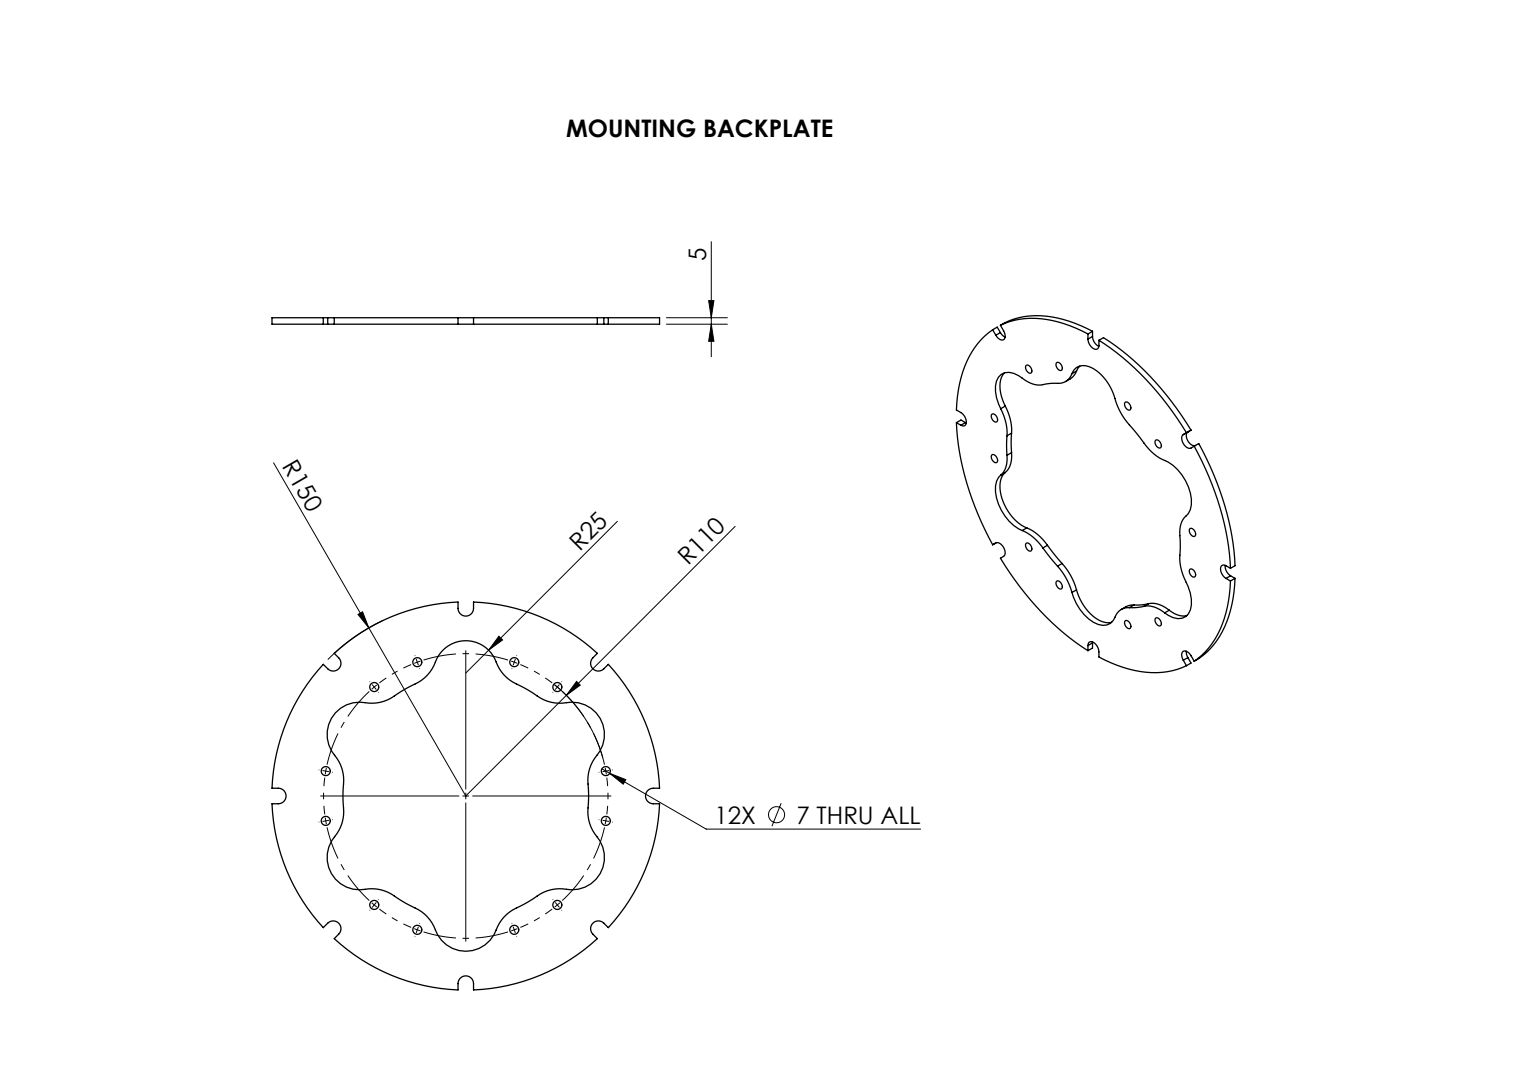
ISO-10303-21;
HEADER;
FILE_DESCRIPTION (('STEP AP214'),
    '1' );
FILE_NAME ('mounting backplate.step',
    '2026-09-21T15:58:29',
    ( '' ),
    ( '' ),
    'SwSTEP 2.0',
    'SolidWorks 2026',
    '' );
FILE_SCHEMA (( 'AUTOMOTIVE_DESIGN' ));
ENDSEC;

DATA;
#3=ORIENTED_EDGE ( 'NONE', *, *, #6672, .T. ) ;
#13=EDGE_CURVE ( 'NONE', #31164, #27343, #2215, .T. ) ;
#22=EDGE_CURVE ( 'NONE', #8678, #8115, #12991, .T. ) ;
#37=CARTESIAN_POINT ( 'NONE',  ( -5.999999999999998224, -145.0000000000000568, 27.50000000000000000 ) ) ;
#40=VERTEX_POINT ( 'NONE', #29073 ) ;
#41=B_SPLINE_CURVE_WITH_KNOTS ( 'NONE', 3,
 ( #1307, #24180, #18746, #30167, #7133, #7874, #14025, #11030, #2597, #10859, #22124, #25848, #25677, #17230, #22672, #5430, #8588, #5792, #22296, #5042, #34557, #25296, #13675, #2430, #10681, #28652, #33922, #25131, #25473, #19674, #2985, #16478, #17025, #14220, #34121 ),
 .UNSPECIFIED., .F., .F.,
 ( 4, 2, 1, 1, 2, 2, 1, 2, 2, 2, 2, 1, 2, 2, 1, 2, 2, 1, 1, 2, 4 ),
 ( 0.05563282717606015532, 0.06778080578355423491, 0.07992878439104830757, 0.1042247416060363280, 0.1163727202135303451, 0.1285206988210243761, 0.1528166560360122717, 0.1771126132510001672, 0.1892605918584941982, 0.2014085704659882570, 0.2500004848959641035, 0.2985923993259401166, 0.3107403779334341754, 0.3228883565409281786, 0.3471843137559161296, 0.3714802709709040252, 0.3836282495783980284, 0.3957762281858920317, 0.4200721854008799272, 0.4322201640083740415, 0.4443681426158681003 ),
 .UNSPECIFIED. ) ;
#42=CARTESIAN_POINT ( 'NONE',  ( -51.68138994340220904, 113.8157894736842053, 27.50000000000000000 ) ) ;
#46=ORIENTED_EDGE ( 'NONE', *, *, #8957, .F. ) ;
#56=DIRECTION ( 'NONE',  ( 1.000000000000000000, 0.000000000000000000, 0.000000000000000000 ) ) ;
#61=FACE_OUTER_BOUND ( 'NONE', #20749, .T. ) ;
#79=DIRECTION ( 'NONE',  ( -0.000000000000000000, -0.000000000000000000, -1.000000000000000000 ) ) ;
#84=FACE_OUTER_BOUND ( 'NONE', #29361, .T. ) ;
#90=DIRECTION ( 'NONE',  ( 0.000000000000000000, 0.000000000000000000, 1.000000000000000000 ) ) ;
#114=VERTEX_POINT ( 'NONE', #394 ) ;
#118=DIRECTION ( 'NONE',  ( -0.7071067811865463515, 0.7071067811865487940, 0.000000000000000000 ) ) ;
#130=ORIENTED_EDGE ( 'NONE', *, *, #1368, .T. ) ;
#139=CARTESIAN_POINT ( 'NONE',  ( 98.28784258492957804, -106.7731239591692116, 32.50000000000000000 ) ) ;
#144=CIRCLE ( 'NONE', #10915, 3.499999999999996003 ) ;
#156=AXIS2_PLACEMENT_3D ( 'NONE', #424, #5891, #17129 ) ;
#188=DIRECTION ( 'NONE',  ( 0.7071067811865512365, 0.7071067811865439090, -0.000000000000000000 ) ) ;
#194=CIRCLE ( 'NONE', #12140, 30.00000000000000000 ) ;
#212=CIRCLE ( 'NONE', #9335, 3.500000000000003109 ) ;
#219=LINE ( 'NONE', #29087, #28624 ) ;
#231=ORIENTED_EDGE ( 'NONE', *, *, #33765, .T. ) ;
#248=ORIENTED_EDGE ( 'NONE', *, *, #1490, .F. ) ;
#250=ORIENTED_EDGE ( 'NONE', *, *, #33993, .T. ) ;
#252=FACE_OUTER_BOUND ( 'NONE', #33217, .T. ) ;
#261=EDGE_CURVE ( 'NONE', #2865, #30153, #36198, .T. ) ;
#273=DIRECTION ( 'NONE',  ( 1.000000000000000000, 0.000000000000000000, 0.000000000000000000 ) ) ;
#277=AXIS2_PLACEMENT_3D ( 'NONE', #26246, #15000, #11980 ) ;
#284=ORIENTED_EDGE ( 'NONE', *, *, #26597, .T. ) ;
#303=DIRECTION ( 'NONE',  ( 0.000000000000000000, 0.000000000000000000, 1.000000000000000000 ) ) ;
#315=ORIENTED_EDGE ( 'NONE', *, *, #9812, .T. ) ;
#343=FILL_AREA_STYLE_COLOUR ( '', #32786 ) ;
#361=CARTESIAN_POINT ( 'NONE',  ( 67.30619744049005249, 84.18124734178236679, 32.50000000000000000 ) ) ;
#375=CARTESIAN_POINT ( 'NONE',  ( -145.0000000000000000, 6.000000000001517009, 32.50000000000000000 ) ) ;
#385=AXIS2_PLACEMENT_3D ( 'NONE', #13978, #33868, #34423 ) ;
#394=CARTESIAN_POINT ( 'NONE',  ( 96.53048327204960799, 102.5304832720492527, 32.50000000000000000 ) ) ;
#412=CARTESIAN_POINT ( 'NONE',  ( -55.27226924886181791, -77.26562141134519379, 27.50000000000000000 ) ) ;
#424=CARTESIAN_POINT ( 'NONE',  ( 0.000000000000000000, 0.000000000000000000, 32.50000000000000000 ) ) ;
#434=CIRCLE ( 'NONE', #22609, 3.500000000000003109 ) ;
#436=CARTESIAN_POINT ( 'NONE',  ( 51.68138994340220904, -113.8157894736842053, 32.50002500000000083 ) ) ;
#440=CARTESIAN_POINT ( 'NONE',  ( -18.19096825468298206, -112.1612438786420256, 32.50000000000000000 ) ) ;
#460=VERTEX_POINT ( 'NONE', #14249 ) ;
#491=CARTESIAN_POINT ( 'NONE',  ( 95.00000000000001421, 0.000000000000000000, 27.50000000000000000 ) ) ;
#492=ORIENTED_EDGE ( 'NONE', *, *, #13456, .T. ) ;
#511=CARTESIAN_POINT ( 'NONE',  ( -6.284666409917640040E-14, -6.000000000000000000, 27.50000000000000000 ) ) ;
#521=AXIS2_PLACEMENT_3D ( 'NONE', #20689, #29495, #32120 ) ;
#525=CARTESIAN_POINT ( 'NONE',  ( 96.53048327204888324, -102.5304832720499633, 27.50000000000000000 ) ) ;
#526=PLANE ( 'NONE',  #25503 ) ;
#527=CARTESIAN_POINT ( 'NONE',  ( 149.8799519615616589, 5.999999999999476863, 32.55002500000000509 ) ) ;
#535=DIRECTION ( 'NONE',  ( 1.000000000000000000, 0.000000000000000000, 0.000000000000000000 ) ) ;
#540=CIRCLE ( 'NONE', #34686, 5.999999999999999112 ) ;
#562=CARTESIAN_POINT ( 'NONE',  ( 82.38629821025696742, 72.56049487126330177, 32.49999999999998579 ) ) ;
#563=DIRECTION ( 'NONE',  ( 0.000000000000000000, 0.000000000000000000, 1.000000000000000000 ) ) ;
#589=FACE_OUTER_BOUND ( 'NONE', #27728, .T. ) ;
#591=ORIENTED_EDGE ( 'NONE', *, *, #22851, .F. ) ;
#613=FACE_OUTER_BOUND ( 'NONE', #23040, .T. ) ;
#615=EDGE_CURVE ( 'NONE', #4570, #3560, #17776, .T. ) ;
#641=CARTESIAN_POINT ( 'NONE',  ( -98.28784258492883907, 106.7731239591698937, 32.50000000000000000 ) ) ;
#643=CYLINDRICAL_SURFACE ( 'NONE', #1498, 30.00000000000000000 ) ;
#646=DIRECTION ( 'NONE',  ( -0.000000000000000000, -0.000000000000000000, 1.000000000000000000 ) ) ;
#653=DIRECTION ( 'NONE',  ( 0.000000000000000000, 0.000000000000000000, 1.000000000000000000 ) ) ;
#654=ADVANCED_FACE ( 'NONE', ( #5002 ), #21520, .F. ) ;
#677=ORIENTED_EDGE ( 'NONE', *, *, #11143, .T. ) ;
#684=EDGE_LOOP ( 'NONE', ( #31991, #3562, #3930, #7996 ) ) ;
#694=CARTESIAN_POINT ( 'NONE',  ( 149.8799519615616589, 5.999999999999476863, 27.50000000000000000 ) ) ;
#711=EDGE_CURVE ( 'NONE', #22882, #22692, #14376, .T. ) ;
#735=CARTESIAN_POINT ( 'NONE',  ( -37.50000000000000000, -103.4105893997321743, 32.50000000000000000 ) ) ;
#738=CARTESIAN_POINT ( 'NONE',  ( 105.8342059669409281, 39.11274920687675660, 32.50000000000000000 ) ) ;
#739=DIRECTION ( 'NONE',  ( 1.000000000000000000, 0.000000000000000000, 0.000000000000000000 ) ) ;
#785=DIRECTION ( 'NONE',  ( -0.000000000000000000, -0.000000000000000000, -1.000000000000000000 ) ) ;
#805=CARTESIAN_POINT ( 'NONE',  ( 2.577124608817066953, -119.9999535335656162, 32.50000000000000000 ) ) ;
#806=EDGE_CURVE ( 'NONE', #8770, #16892, #29355, .T. ) ;
#812=EDGE_CURVE ( 'NONE', #10608, #13259, #17726, .T. ) ;
#813=CYLINDRICAL_SURFACE ( 'NONE', #32755, 30.00000000000000000 ) ;
#815=CARTESIAN_POINT ( 'NONE',  ( -23.49188638668713480, -103.5527587461262442, 32.50001250000000397 ) ) ;
#839=ORIENTED_EDGE ( 'NONE', *, *, #21442, .F. ) ;
#843=PLANE ( 'NONE',  #24821 ) ;
#844=FACE_OUTER_BOUND ( 'NONE', #14924, .T. ) ;
#868=VECTOR ( 'NONE', #29592, 1000.000000000000000 ) ;
#877=CARTESIAN_POINT ( 'NONE',  ( -72.72667006429185221, -101.6652913307173662, 27.50000000000000000 ) ) ;
#891=CARTESIAN_POINT ( 'NONE',  ( -51.68138994340220904, -113.8157894736842053, 32.50002500000000083 ) ) ;
#901=CARTESIAN_POINT ( 'NONE',  ( -94.55012560584668790, 9.234378588655390629, 27.50000000000000000 ) ) ;
#935=ORIENTED_EDGE ( 'NONE', *, *, #19624, .F. ) ;
#938=LINE ( 'NONE', #12358, #6254 ) ;
#941=DIRECTION ( 'NONE',  ( 0.000000000000000000, 0.000000000000000000, 1.000000000000000000 ) ) ;
#963=EDGE_LOOP ( 'NONE', ( #4579, #25349, #35849, #2137 ) ) ;
#976=CYLINDRICAL_SURFACE ( 'NONE', #1827, 3.500000000000003109 ) ;
#986=AXIS2_PLACEMENT_3D ( 'NONE', #19892, #19180, #30599 ) ;
#991=DIRECTION ( 'NONE',  ( 0.000000000000000000, 0.000000000000000000, 1.000000000000000000 ) ) ;
#1012=DIRECTION ( 'NONE',  ( -1.000000000000000000, 0.000000000000000000, 0.000000000000000000 ) ) ;
#1026=VECTOR ( 'NONE', #13351, 1000.000000000000000 ) ;
#1033=LINE ( 'NONE', #12458, #22337 ) ;
#1070=ORIENTED_EDGE ( 'NONE', *, *, #28796, .T. ) ;
#1078=DIRECTION ( 'NONE',  ( 1.000000000000000000, 0.000000000000000000, 0.000000000000000000 ) ) ;
#1080=AXIS2_PLACEMENT_3D ( 'NONE', #23094, #15030, #8849 ) ;
#1098=ORIENTED_EDGE ( 'NONE', *, *, #4957, .T. ) ;
#1100=DIRECTION ( 'NONE',  ( 0.000000000000000000, 0.000000000000000000, 1.000000000000000000 ) ) ;
#1122=CARTESIAN_POINT ( 'NONE',  ( 97.20669606277387231, 67.55917549538906997, 32.49999999999999289 ) ) ;
#1124=CIRCLE ( 'NONE', #13086, 95.00000000000001421 ) ;
#1164=CARTESIAN_POINT ( 'NONE',  ( 4.242640687119292764, 4.242640687119187071, 27.50000000000000000 ) ) ;
#1188=EDGE_LOOP ( 'NONE', ( #33444, #30548, #5664, #10870 ) ) ;
#1196=CYLINDRICAL_SURFACE ( 'NONE', #14748, 3.500000000000003109 ) ;
#1209=ORIENTED_EDGE ( 'NONE', *, *, #23387, .T. ) ;
#1214=CARTESIAN_POINT ( 'NONE',  ( -4.242640687119273224, -4.242640687119226151, 32.50000000000000000 ) ) ;
#1215=VECTOR ( 'NONE', #21555, 1000.000000000000000 ) ;
#1224=VERTEX_POINT ( 'NONE', #20518 ) ;
#1233=DIRECTION ( 'NONE',  ( 1.000000000000000000, 0.000000000000000000, 0.000000000000000000 ) ) ;
#1238=ORIENTED_EDGE ( 'NONE', *, *, #28621, .T. ) ;
#1262=CARTESIAN_POINT ( 'NONE',  ( 0.000000000000000000, 95.00000000000001421, 32.50000000000000000 ) ) ;
#1293=CARTESIAN_POINT ( 'NONE',  ( 51.68138994340220904, 113.8157894736842053, 27.50000000000000000 ) ) ;
#1294=AXIS2_PLACEMENT_3D ( 'NONE', #11887, #20153, #8708 ) ;
#1297=EDGE_LOOP ( 'NONE', ( #315, #8437, #30494, #23979 ) ) ;
#1305=DIRECTION ( 'NONE',  ( 0.000000000000000000, 0.000000000000000000, 1.000000000000000000 ) ) ;
#1307=CARTESIAN_POINT ( 'NONE',  ( 101.4252494179806661, -31.43181965332042438, 32.50001250000000397 ) ) ;
#1308=CARTESIAN_POINT ( 'NONE',  ( -37.50000000000000000, 103.4105893997321743, 32.50000000000000000 ) ) ;
#1355=DIRECTION ( 'NONE',  ( -0.000000000000000000, -0.000000000000000000, -1.000000000000000000 ) ) ;
#1358=VERTEX_POINT ( 'NONE', #15276 ) ;
#1368=EDGE_CURVE ( 'NONE', #28369, #25631, #212, .T. ) ;
#1381=CARTESIAN_POINT ( 'NONE',  ( 124.4080600076931375, 12.15049814296589226, 32.50000000000000000 ) ) ;
#1388=DIRECTION ( 'NONE',  ( -1.000000000000000000, 0.000000000000000000, 0.000000000000000000 ) ) ;
#1391=EDGE_CURVE ( 'NONE', #4682, #26755, #18090, .T. ) ;
#1398=ORIENTED_EDGE ( 'NONE', *, *, #1368, .F. ) ;
#1400=DIRECTION ( 'NONE',  ( -0.000000000000000000, -0.000000000000000000, 1.000000000000000000 ) ) ;
#1403=EDGE_CURVE ( 'NONE', #8057, #11432, #1033, .T. ) ;
#1422=PRODUCT_CONTEXT ( 'NONE', #17085, 'mechanical' ) ;
#1429=DIRECTION ( 'NONE',  ( 0.000000000000000000, 0.000000000000000000, 1.000000000000000000 ) ) ;
#1442=VERTEX_POINT ( 'NONE', #16390 ) ;
#1456=CIRCLE ( 'NONE', #277, 3.499999999999996003 ) ;
#1458=EDGE_LOOP ( 'NONE', ( #32965, #6091, #32772, #35012 ) ) ;
#1490=EDGE_CURVE ( 'NONE', #35726, #27793, #15131, .T. ) ;
#1498=AXIS2_PLACEMENT_3D ( 'NONE', #17511, #11883, #32492 ) ;
#1567=EDGE_CURVE ( 'NONE', #4390, #26755, #33266, .T. ) ;
#1589=CYLINDRICAL_SURFACE ( 'NONE', #32182, 3.500000000000003109 ) ;
#1598=VERTEX_POINT ( 'NONE', #5514 ) ;
#1604=CARTESIAN_POINT ( 'NONE',  ( -108.3061974404900241, -19.22934205794863516, 27.50000000000000000 ) ) ;
#1605=CARTESIAN_POINT ( 'NONE',  ( 4.242640687119310527, 4.242640687119267007, 32.50000000000000000 ) ) ;
#1607=EDGE_CURVE ( 'NONE', #14541, #13732, #10344, .T. ) ;
#1609=FACE_OUTER_BOUND ( 'NONE', #3806, .T. ) ;
#1613=DIRECTION ( 'NONE',  ( 1.000000000000000000, 0.000000000000000000, 0.000000000000000000 ) ) ;
#1617=CARTESIAN_POINT ( 'NONE',  ( 101.7384897088151234, 110.2237710830533217, 32.50000000000000000 ) ) ;
#1624=ORIENTED_EDGE ( 'NONE', *, *, #19700, .T. ) ;
#1636=ADVANCED_FACE ( 'NONE', ( #19937 ), #2690, .F. ) ;
#1641=AXIS2_PLACEMENT_3D ( 'NONE', #16254, #4438, #15690 ) ;
#1643=ORIENTED_EDGE ( 'NONE', *, *, #12876, .F. ) ;
#1657=ORIENTED_EDGE ( 'NONE', *, *, #3901, .F. ) ;
#1660=AXIS2_PLACEMENT_3D ( 'NONE', #17232, #31452, #28655 ) ;
#1661=LINE ( 'NONE', #35609, #19441 ) ;
#1667=CARTESIAN_POINT ( 'NONE',  ( -107.0891125874437506, 43.89216747908891136, 32.49999999999999289 ) ) ;
#1673=LINE ( 'NONE', #26984, #868 ) ;
#1677=AXIS2_PLACEMENT_3D ( 'NONE', #27123, #4086, #26955 ) ;
#1692=ORIENTED_EDGE ( 'NONE', *, *, #6728, .T. ) ;
#1706=AXIS2_PLACEMENT_3D ( 'NONE', #9005, #11439, #32023 ) ;
#1712=CARTESIAN_POINT ( 'NONE',  ( -67.30619744049063513, -84.18124734178186941, 27.50000000000000000 ) ) ;
#1739=CARTESIAN_POINT ( 'NONE',  ( -103.1837590831665210, -33.77668192579397299, 32.49999999999999289 ) ) ;
#1760=DIRECTION ( 'NONE',  ( -0.000000000000000000, -0.000000000000000000, -1.000000000000000000 ) ) ;
#1767=ORIENTED_EDGE ( 'NONE', *, *, #6528, .F. ) ;
#1768=CYLINDRICAL_SURFACE ( 'NONE', #23835, 95.00000000000001421 ) ;
#1784=ORIENTED_EDGE ( 'NONE', *, *, #22476, .T. ) ;
#1786=CARTESIAN_POINT ( 'NONE',  ( -145.0000000000000568, 1.518182058997189877E-12, 32.55002500000000509 ) ) ;
#1787=CARTESIAN_POINT ( 'NONE',  ( 145.0000000000000568, -5.056524707326808249E-13, 32.55002500000000509 ) ) ;
#1809=FACE_OUTER_BOUND ( 'NONE', #29343, .T. ) ;
#1827=AXIS2_PLACEMENT_3D ( 'NONE', #29849, #8087, #1908 ) ;
#1830=CARTESIAN_POINT ( 'NONE',  ( 0.000000000000000000, -95.00000000000001421, 32.50002500000000083 ) ) ;
#1831=CARTESIAN_POINT ( 'NONE',  ( -103.1654841881149025, 61.26096253783315859, 32.50000000000000711 ) ) ;
#1880=ORIENTED_EDGE ( 'NONE', *, *, #6661, .F. ) ;
#1908=DIRECTION ( 'NONE',  ( 1.000000000000000000, 0.000000000000000000, 0.000000000000000000 ) ) ;
#1918=CARTESIAN_POINT ( 'NONE',  ( -107.2777853369584591, -46.05195005975305378, 32.50000000000000000 ) ) ;
#1920=EDGE_LOOP ( 'NONE', ( #8732, #36744, #26794, #12307, #11729, #24164, #19809, #10074, #25151, #33826, #24025, #21911, #12744, #33055, #6237, #10358, #21105, #28122, #28960, #16884, #3124, #8179, #36525, #19792, #28859, #18087, #7295, #250, #22492, #26605, #15987, #18220, #231, #15241, #9497 ) ) ;
#1924=FACE_OUTER_BOUND ( 'NONE', #9242, .T. ) ;
#1932=DIRECTION ( 'NONE',  ( -0.000000000000000000, -0.000000000000000000, -1.000000000000000000 ) ) ;
#1946=VERTEX_POINT ( 'NONE', #36374 ) ;
#1950=EDGE_CURVE ( 'NONE', #13345, #8665, #9606, .T. ) ;
#1952=VERTEX_POINT ( 'NONE', #25297 ) ;
#1961=EDGE_CURVE ( 'NONE', #22389, #3923, #34473, .T. ) ;
#1962=AXIS2_PLACEMENT_3D ( 'NONE', #32236, #34705, #9006 ) ;
#1963=DIRECTION ( 'NONE',  ( 0.000000000000000000, 0.000000000000000000, 1.000000000000000000 ) ) ;
#1972=ADVANCED_FACE ( 'NONE', ( #8779 ), #526, .F. ) ;
#1973=ORIENTED_EDGE ( 'NONE', *, *, #6672, .F. ) ;
#1992=CARTESIAN_POINT ( 'NONE',  ( -111.8061974404900241, -19.22934205794863516, 27.50000000000000000 ) ) ;
#1998=EDGE_CURVE ( 'NONE', #114, #35512, #32055, .T. ) ;
#2006=EDGE_CURVE ( 'NONE', #23321, #6715, #20562, .T. ) ;
#2025=CARTESIAN_POINT ( 'NONE',  ( 72.72667006429044534, -101.6652913307183610, 32.50000000000000000 ) ) ;
#2031=ADVANCED_FACE ( 'NONE', ( #34470 ), #14967, .F. ) ;
#2033=EDGE_LOOP ( 'NONE', ( #19508, #14993, #29571, #36394 ) ) ;
#2049=VERTEX_POINT ( 'NONE', #139 ) ;
#2070=CARTESIAN_POINT ( 'NONE',  ( 23.49154088336464952, -103.5526315789473699, 32.50002500000000083 ) ) ;
#2085=EDGE_CURVE ( 'NONE', #19856, #15010, #11705, .T. ) ;
#2093=CARTESIAN_POINT ( 'NONE',  ( -82.27241335952211898, -47.49999999999924682, 27.50000000000000000 ) ) ;
#2113=LINE ( 'NONE', #10758, #18957 ) ;
#2118=EDGE_LOOP ( 'NONE', ( #28713, #23285, #17247, #29365 ) ) ;
#2119=CARTESIAN_POINT ( 'NONE',  ( 0.000000000000000000, 0.000000000000000000, 27.50000000000000000 ) ) ;
#2126=CIRCLE ( 'NONE', #33260, 30.00000000000001421 ) ;
#2133=CARTESIAN_POINT ( 'NONE',  ( 0.000000000000000000, 0.000000000000000000, 27.50000000000000000 ) ) ;
#2137=ORIENTED_EDGE ( 'NONE', *, *, #34736, .T. ) ;
#2155=DIRECTION ( 'NONE',  ( 0.000000000000000000, 0.000000000000000000, 1.000000000000000000 ) ) ;
#2160=FACE_OUTER_BOUND ( 'NONE', #24834, .T. ) ;
#2184=ORIENTED_EDGE ( 'NONE', *, *, #13444, .F. ) ;
#2203=ORIENTED_EDGE ( 'NONE', *, *, #22583, .F. ) ;
#2212=VECTOR ( 'NONE', #29599, 1000.000000000000000 ) ;
#2215=CIRCLE ( 'NONE', #13591, 30.00000000000000000 ) ;
#2219=ADVANCED_FACE ( 'NONE', ( #84 ), #813, .T. ) ;
#2229=CARTESIAN_POINT ( 'NONE',  ( 39.27785635698568711, -86.50000000000001421, 27.50000000000000000 ) ) ;
#2235=DIRECTION ( 'NONE',  ( -0.000000000000000000, -0.000000000000000000, -1.000000000000000000 ) ) ;
#2238=CARTESIAN_POINT ( 'NONE',  ( 70.80619744048946984, -84.18124734178287838, 32.50000000000000000 ) ) ;
#2244=ORIENTED_EDGE ( 'NONE', *, *, #12311, .T. ) ;
#2256=ORIENTED_EDGE ( 'NONE', *, *, #35923, .T. ) ;
#2271=ADVANCED_FACE ( 'NONE', ( #29754 ), #12868, .F. ) ;
#2280=DIRECTION ( 'NONE',  ( 0.000000000000000000, 0.000000000000000000, 1.000000000000000000 ) ) ;
#2283=LINE ( 'NONE', #13718, #34971 ) ;
#2351=CARTESIAN_POINT ( 'NONE',  ( -70.80619744049063513, -84.18124734178186941, 32.50000000000000000 ) ) ;
#2360=CARTESIAN_POINT ( 'NONE',  ( 74.30619744049005249, 84.18124734178236679, 32.50000000000000000 ) ) ;
#2364=CARTESIAN_POINT ( 'NONE',  ( 124.4080600076931375, 12.15049814296589226, 27.50000000000000000 ) ) ;
#2366=EDGE_CURVE ( 'NONE', #3923, #5373, #33322, .T. ) ;
#2374=DIRECTION ( 'NONE',  ( 1.000000000000000000, 0.000000000000000000, 0.000000000000000000 ) ) ;
#2397=EDGE_LOOP ( 'NONE', ( #7938, #25080, #6315, #13329 ) ) ;
#2425=CYLINDRICAL_SURFACE ( 'NONE', #4963, 5.999999999999999112 ) ;
#2427=DIRECTION ( 'NONE',  ( 1.000000000000000000, 0.000000000000000000, 0.000000000000000000 ) ) ;
#2430=CARTESIAN_POINT ( 'NONE',  ( 95.09707527045419795, -69.00156695264264783, 32.50000000000000000 ) ) ;
#2440=DIRECTION ( 'NONE',  ( 0.000000000000000000, 0.000000000000000000, 1.000000000000000000 ) ) ;
#2443=PRODUCT_DEFINITION_CONTEXT ( 'detailed design', #24048, 'design' ) ;
#2451=SHAPE_REPRESENTATION_RELATIONSHIP ( 'NONE' , 'NONE' ,  #6396, #29583 ) ;
#2481=CARTESIAN_POINT ( 'NONE',  ( -107.2742747693529566, -47.50000423952285900, 32.50001250000000397 ) ) ;
#2495=ORIENTED_EDGE ( 'NONE', *, *, #29664, .F. ) ;
#2497=LINE ( 'NONE', #7564, #32093 ) ;
#2537=DIRECTION ( 'NONE',  ( 1.000000000000000000, 0.000000000000000000, 0.000000000000000000 ) ) ;
#2551=AXIS2_PLACEMENT_3D ( 'NONE', #7357, #27038, #35675 ) ;
#2566=ADVANCED_FACE ( 'NONE', ( #35925 ), #10231, .F. ) ;
#2570=CARTESIAN_POINT ( 'NONE',  ( -34.00000000000000000, 103.4105893997321743, 27.50000000000000000 ) ) ;
#2571=ORIENTED_EDGE ( 'NONE', *, *, #21867, .F. ) ;
#2597=CARTESIAN_POINT ( 'NONE',  ( 106.4067760678514958, -40.94775080679610113, 32.50000000000000711 ) ) ;
#2598=CARTESIAN_POINT ( 'NONE',  ( -99.75141825464123713, -65.47128713877522443, 32.50000000000000000 ) ) ;
#2606=CYLINDRICAL_SURFACE ( 'NONE', #25353, 6.000000000000005329 ) ;
#2614=VERTEX_POINT ( 'NONE', #7042 ) ;
#2633=DIRECTION ( 'NONE',  ( 1.000000000000000000, 0.000000000000000000, 0.000000000000000000 ) ) ;
#2646=PLANE ( 'NONE',  #20611 ) ;
#2649=CARTESIAN_POINT ( 'NONE',  ( 77.93343913441695747, 72.12058696850802164, 32.50002500000000083 ) ) ;
#2654=CARTESIAN_POINT ( 'NONE',  ( 94.55012560584674475, -9.234378588654731601, 27.50000000000000000 ) ) ;
#2658=CARTESIAN_POINT ( 'NONE',  ( 70.80619744048946984, -84.18124734178287838, 27.50000000000000000 ) ) ;
#2661=ADVANCED_FACE ( 'NONE', ( #844 ), #4240, .F. ) ;
#2682=AXIS2_PLACEMENT_3D ( 'NONE', #8607, #28477, #3553 ) ;
#2683=CARTESIAN_POINT ( 'NONE',  ( -9.944410904869345202, 118.0778278770615657, 27.49998800000000188 ) ) ;
#2690=CYLINDRICAL_SURFACE ( 'NONE', #13192, 3.499999999999996003 ) ;
#2692=EDGE_LOOP ( 'NONE', ( #2950, #18707 ) ) ;
#2709=EDGE_CURVE ( 'NONE', #33855, #4390, #8146, .T. ) ;
#2715=DIRECTION ( 'NONE',  ( 0.7071067811865563435, 0.7071067811865388020, 0.000000000000000000 ) ) ;
#2718=AXIS2_PLACEMENT_3D ( 'NONE', #2364, #13801, #11345 ) ;
#2720=DIRECTION ( 'NONE',  ( 0.000000000000000000, 0.000000000000000000, 1.000000000000000000 ) ) ;
#2728=VECTOR ( 'NONE', #33700, 1000.000000000000000 ) ;
#2734=EDGE_LOOP ( 'NONE', ( #28020, #1692 ) ) ;
#2735=CARTESIAN_POINT ( 'NONE',  ( 0.000000000000000000, 0.000000000000000000, 27.50000000000000000 ) ) ;
#2738=CIRCLE ( 'NONE', #15310, 3.500000000000003109 ) ;
#2782=ORIENTED_EDGE ( 'NONE', *, *, #13290, .T. ) ;
#2783=ADVANCED_FACE ( 'NONE', ( #13780 ), #25225, .F. ) ;
#2785=DIRECTION ( 'NONE',  ( -1.000000000000000000, 0.000000000000000000, 0.000000000000000000 ) ) ;
#2786=AXIS2_PLACEMENT_3D ( 'NONE', #8512, #5695, #37026 ) ;
#2794=DIRECTION ( 'NONE',  ( -0.000000000000000000, -0.000000000000000000, 1.000000000000000000 ) ) ;
#2818=AXIS2_PLACEMENT_3D ( 'NONE', #7218, #35711, #20701 ) ;
#2820=ORIENTED_EDGE ( 'NONE', *, *, #34666, .F. ) ;
#2822=ORIENTED_EDGE ( 'NONE', *, *, #34666, .T. ) ;
#2826=ORIENTED_EDGE ( 'NONE', *, *, #22046, .F. ) ;
#2833=DIRECTION ( 'NONE',  ( 0.000000000000000000, 0.000000000000000000, 1.000000000000000000 ) ) ;
#2853=LINE ( 'NONE', #14628, #25274 ) ;
#2861=VECTOR ( 'NONE', #23326, 1000.000000000000000 ) ;
#2865=VERTEX_POINT ( 'NONE', #8347 ) ;
#2880=EDGE_CURVE ( 'NONE', #13349, #22389, #194, .T. ) ;
#2884=AXIS2_PLACEMENT_3D ( 'NONE', #29890, #32693, #10016 ) ;
#2885=CARTESIAN_POINT ( 'NONE',  ( 37.50000000000000000, 103.4105893997321743, 27.50000000000000000 ) ) ;
#2923=DIRECTION ( 'NONE',  ( 1.000000000000000000, 0.000000000000000000, 0.000000000000000000 ) ) ;
#2927=CARTESIAN_POINT ( 'NONE',  ( 70.80619744049005249, 84.18124734178236679, 27.50000000000000000 ) ) ;
#2950=ORIENTED_EDGE ( 'NONE', *, *, #29826, .T. ) ;
#2985=CARTESIAN_POINT ( 'NONE',  ( 82.38669124558430212, -72.56045967525361107, 32.50000000000000000 ) ) ;
#2990=ORIENTED_EDGE ( 'NONE', *, *, #23402, .T. ) ;
#2991=ORIENTED_EDGE ( 'NONE', *, *, #28888, .T. ) ;
#3007=CARTESIAN_POINT ( 'NONE',  ( 101.7384897088151234, 110.2237710830533217, 27.50000000000000000 ) ) ;
#3013=VERTEX_POINT ( 'NONE', #29862 ) ;
#3019=EDGE_CURVE ( 'NONE', #6052, #11631, #26874, .T. ) ;
#3020=AXIS2_PLACEMENT_3D ( 'NONE', #10419, #29933, #12849 ) ;
#3035=EDGE_CURVE ( 'NONE', #17786, #28544, #21425, .T. ) ;
#3062=LINE ( 'NONE', #31183, #7099 ) ;
#3070=DIRECTION ( 'NONE',  ( 1.000000000000000000, 0.000000000000000000, 0.000000000000000000 ) ) ;
#3089=DIRECTION ( 'NONE',  ( -0.000000000000000000, -0.000000000000000000, -1.000000000000000000 ) ) ;
#3098=LINE ( 'NONE', #26149, #15179 ) ;
#3124=ORIENTED_EDGE ( 'NONE', *, *, #35306, .F. ) ;
#3138=ORIENTED_EDGE ( 'NONE', *, *, #34210, .T. ) ;
#3168=( NAMED_UNIT ( * ) SI_UNIT ( $, .STERADIAN. ) SOLID_ANGLE_UNIT ( ) );
#3196=DIRECTION ( 'NONE',  ( -0.7071067811865439090, 0.7071067811865512365, 0.000000000000000000 ) ) ;
#3206=EDGE_CURVE ( 'NONE', #29329, #27821, #36748, .T. ) ;
#3207=ORIENTED_EDGE ( 'NONE', *, *, #13498, .F. ) ;
#3208=EDGE_CURVE ( 'NONE', #25631, #28369, #4420, .T. ) ;
#3210=ORIENTED_EDGE ( 'NONE', *, *, #13181, .F. ) ;
#3217=ORIENTED_EDGE ( 'NONE', *, *, #9460, .T. ) ;
#3229=DIRECTION ( 'NONE',  ( -0.000000000000000000, -0.000000000000000000, -1.000000000000000000 ) ) ;
#3233=EDGE_CURVE ( 'NONE', #460, #28766, #28711, .T. ) ;
#3248=CIRCLE ( 'NONE', #30778, 6.000000000000005329 ) ;
#3255=CARTESIAN_POINT ( 'NONE',  ( 5.078940004773329520, -119.6165172753982375, 32.50000000000000000 ) ) ;
#3256=AXIS2_PLACEMENT_3D ( 'NONE', #18164, #15733, #27155 ) ;
#3269=EDGE_LOOP ( 'NONE', ( #17380, #35791, #20188, #31378 ) ) ;
#3306=ORIENTED_EDGE ( 'NONE', *, *, #16688, .F. ) ;
#3313=EDGE_CURVE ( 'NONE', #8115, #13345, #2853, .T. ) ;
#3321=CIRCLE ( 'NONE', #15906, 24.99999999999999289 ) ;
#3331=CARTESIAN_POINT ( 'NONE',  ( 6.000000000000000000, 0.000000000000000000, 27.50000000000000000 ) ) ;
#3337=VECTOR ( 'NONE', #35736, 1000.000000000000000 ) ;
#3374=CARTESIAN_POINT ( 'NONE',  ( 107.3056475171454593, 47.85569953350209715, 32.50000000000000000 ) ) ;
#3381=DIRECTION ( 'NONE',  ( 0.000000000000000000, 0.000000000000000000, 1.000000000000000000 ) ) ;
#3396=AXIS2_PLACEMENT_3D ( 'NONE', #12624, #4011, #30237 ) ;
#3423=LINE ( 'NONE', #25868, #29850 ) ;
#3429=VECTOR ( 'NONE', #5045, 1000.000000000000114 ) ;
#3431=CYLINDRICAL_SURFACE ( 'NONE', #31338, 24.99999999999999289 ) ;
#3446=CARTESIAN_POINT ( 'NONE',  ( 124.4080600076930665, -12.15049814296675201, 32.50002500000000083 ) ) ;
#3454=CARTESIAN_POINT ( 'NONE',  ( -21.64585576624245888, -107.6291973900578398, 32.50000000000000000 ) ) ;
#3455=VERTEX_POINT ( 'NONE', #3587 ) ;
#3457=VERTEX_POINT ( 'NONE', #9581 ) ;
#3461=CYLINDRICAL_SURFACE ( 'NONE', #11780, 3.500000000000003109 ) ;
#3468=DIRECTION ( 'NONE',  ( -0.000000000000000000, -0.000000000000000000, 1.000000000000000000 ) ) ;
#3474=ORIENTED_EDGE ( 'NONE', *, *, #27292, .F. ) ;
#3480=VECTOR ( 'NONE', #24309, 1000.000000000000000 ) ;
#3487=CARTESIAN_POINT ( 'NONE',  ( 70.80619744049005249, 84.18124734178236679, 27.50000000000000000 ) ) ;
#3501=EDGE_LOOP ( 'NONE', ( #18075, #4481 ) ) ;
#3525=ORIENTED_EDGE ( 'NONE', *, *, #10328, .F. ) ;
#3528=ORIENTED_EDGE ( 'NONE', *, *, #26953, .F. ) ;
#3532=CARTESIAN_POINT ( 'NONE',  ( 39.27785635698568711, 86.50000000000001421, 32.50000000000000000 ) ) ;
#3535=CARTESIAN_POINT ( 'NONE',  ( 70.80619744048946984, -84.18124734178287838, 32.50000000000000000 ) ) ;
#3536=DIRECTION ( 'NONE',  ( -0.000000000000000000, -0.000000000000000000, -1.000000000000000000 ) ) ;
#3545=FACE_OUTER_BOUND ( 'NONE', #15002, .T. ) ;
#3553=DIRECTION ( 'NONE',  ( 1.000000000000000000, 0.000000000000000000, 0.000000000000000000 ) ) ;
#3560=VERTEX_POINT ( 'NONE', #24388 ) ;
#3562=ORIENTED_EDGE ( 'NONE', *, *, #1567, .T. ) ;
#3570=CARTESIAN_POINT ( 'NONE',  ( 92.89147506197157611, 70.24558514894413008, 32.49999999999999289 ) ) ;
#3571=FACE_OUTER_BOUND ( 'NONE', #9966, .T. ) ;
#3587=CARTESIAN_POINT ( 'NONE',  ( -110.2237710830543733, -101.7384897088139724, 32.50000000000000000 ) ) ;
#3588=DIRECTION ( 'NONE',  ( -0.000000000000000000, -0.000000000000000000, 1.000000000000000000 ) ) ;
#3596=AXIS2_PLACEMENT_3D ( 'NONE', #15212, #33026, #3969 ) ;
#3630=CARTESIAN_POINT ( 'NONE',  ( 101.7384897088151234, 110.2237710830533217, 32.55002500000000509 ) ) ;
#3637=CARTESIAN_POINT ( 'NONE',  ( -8.711298609632770251, -118.4422998056053160, 32.50000000000000000 ) ) ;
#3640=ORIENTED_EDGE ( 'NONE', *, *, #12272, .F. ) ;
#3655=CARTESIAN_POINT ( 'NONE',  ( 96.53048327204960799, 102.5304832720492527, 27.50000000000000000 ) ) ;
#3658=CARTESIAN_POINT ( 'NONE',  ( 6.123233995736731770E-16, -145.0000000000000568, 27.50000000000000000 ) ) ;
#3659=CARTESIAN_POINT ( 'NONE',  ( -82.27241335952113843, 47.50000000000096634, 32.50002500000000083 ) ) ;
#3694=VERTEX_POINT ( 'NONE', #22861 ) ;
#3700=EDGE_LOOP ( 'NONE', ( #1070, #30331 ) ) ;
#3712=CARTESIAN_POINT ( 'NONE',  ( 102.5304832720496080, 102.5304832720492527, 32.50000000000000000 ) ) ;
#3740=CARTESIAN_POINT ( 'NONE',  ( 105.2117281555539705, 57.76803422138092259, 32.50000000000000711 ) ) ;
#3749=CARTESIAN_POINT ( 'NONE',  ( 55.27226924886075921, -77.26562141134597539, 32.50000000000000000 ) ) ;
#3756=DIRECTION ( 'NONE',  ( 1.000000000000000000, 0.000000000000000000, 0.000000000000000000 ) ) ;
#3763=EDGE_CURVE ( 'NONE', #3694, #34519, #5253, .T. ) ;
#3770=CARTESIAN_POINT ( 'NONE',  ( 70.80619744049005249, 84.18124734178236679, 32.50000000000000000 ) ) ;
#3789=VERTEX_POINT ( 'NONE', #36923 ) ;
#3794=DIRECTION ( 'NONE',  ( 0.000000000000000000, 0.000000000000000000, 1.000000000000000000 ) ) ;
#3803=CARTESIAN_POINT ( 'NONE',  ( -20.26379314223832395, -109.7460900736713540, 32.49999999999999289 ) ) ;
#3806=EDGE_LOOP ( 'NONE', ( #1209, #3217, #5314, #6545 ) ) ;
#3824=CARTESIAN_POINT ( 'NONE',  ( 0.000000000000000000, 0.000000000000000000, 27.50000000000000000 ) ) ;
#3825=DIRECTION ( 'NONE',  ( -0.000000000000000000, -0.000000000000000000, 1.000000000000000000 ) ) ;
#3827=CARTESIAN_POINT ( 'NONE',  ( -5.999999999999998224, -145.0000000000000568, 32.55002500000000509 ) ) ;
#3828=CIRCLE ( 'NONE', #22403, 30.00000000000001421 ) ;
#3829=CARTESIAN_POINT ( 'NONE',  ( 101.7384897088143560, -110.2237710830540180, 27.50000000000000000 ) ) ;
#3846=CARTESIAN_POINT ( 'NONE',  ( 149.8799519615616020, -6.000000000000508038, 32.55002500000000509 ) ) ;
#3849=CARTESIAN_POINT ( 'NONE',  ( 55.27226924886075921, -77.26562141134598960, 27.50000000000000000 ) ) ;
#3866=CARTESIAN_POINT ( 'NONE',  ( 72.72667006429115588, 101.6652913307178636, 27.50000000000000000 ) ) ;
#3878=CARTESIAN_POINT ( 'NONE',  ( 0.000000000000000000, 0.000000000000000000, 27.50000000000000000 ) ) ;
#3888=AXIS2_PLACEMENT_3D ( 'NONE', #9689, #20733, #32170 ) ;
#3889=FACE_OUTER_BOUND ( 'NONE', #31067, .T. ) ;
#3893=ORIENTED_EDGE ( 'NONE', *, *, #812, .F. ) ;
#3901=EDGE_CURVE ( 'NONE', #30601, #1442, #34110, .T. ) ;
#3916=DIRECTION ( 'NONE',  ( 3.554796214472773777E-16, 1.000000000000000000, 0.000000000000000000 ) ) ;
#3920=CARTESIAN_POINT ( 'NONE',  ( 77.93337901593585570, 72.12093275448846441, 32.50001250000000397 ) ) ;
#3923=VERTEX_POINT ( 'NONE', #12469 ) ;
#3925=LINE ( 'NONE', #9924, #26641 ) ;
#3930=ORIENTED_EDGE ( 'NONE', *, *, #1391, .F. ) ;
#3962=ADVANCED_FACE ( 'NONE', ( #8149 ), #22391, .F. ) ;
#3969=DIRECTION ( 'NONE',  ( 1.000000000000000000, 0.000000000000000000, 0.000000000000000000 ) ) ;
#4011=DIRECTION ( 'NONE',  ( -0.000000000000000000, 0.000000000000000000, -1.000000000000000000 ) ) ;
#4036=ORIENTED_EDGE ( 'NONE', *, *, #5338, .F. ) ;
#4068=CARTESIAN_POINT ( 'NONE',  ( -104.8061974404900241, -19.22934205794863516, 27.50000000000000000 ) ) ;
#4081=CYLINDRICAL_SURFACE ( 'NONE', #20150, 25.00000000000000000 ) ;
#4086=DIRECTION ( 'NONE',  ( -1.000000000000000000, 3.554796214472773777E-16, 0.000000000000000000 ) ) ;
#4100=ORIENTED_EDGE ( 'NONE', *, *, #1961, .F. ) ;
#4116=VECTOR ( 'NONE', #646, 1000.000000000000000 ) ;
#4137=LINE ( 'NONE', #21179, #7117 ) ;
#4141=ORIENTED_EDGE ( 'NONE', *, *, #22583, .T. ) ;
#4175=EDGE_CURVE ( 'NONE', #5373, #13276, #26278, .T. ) ;
#4210=ORIENTED_EDGE ( 'NONE', *, *, #27786, .T. ) ;
#4214=AXIS2_PLACEMENT_3D ( 'NONE', #6445, #17885, #23688 ) ;
#4221=DIRECTION ( 'NONE',  ( -0.000000000000000000, 0.000000000000000000, -1.000000000000000000 ) ) ;
#4223=CIRCLE ( 'NONE', #34762, 150.0000000000000284 ) ;
#4240=CYLINDRICAL_SURFACE ( 'NONE', #35229, 3.500000000000003109 ) ;
#4253=PLANE ( 'NONE',  #22465 ) ;
#4270=CARTESIAN_POINT ( 'NONE',  ( 67.30619744048945563, -84.18124734178287838, 32.50000000000000000 ) ) ;
#4272=ADVANCED_FACE ( 'NONE', ( #8693 ), #31559, .T. ) ;
#4276=CARTESIAN_POINT ( 'NONE',  ( -104.1069301565558050, 59.68452040699722261, 32.50000000000000000 ) ) ;
#4310=VERTEX_POINT ( 'NONE', #35686 ) ;
#4331=ADVANCED_FACE ( 'NONE', ( #32482 ), #21232, .F. ) ;
#4361=DIRECTION ( 'NONE',  ( 1.000000000000000000, 0.000000000000000000, 0.000000000000000000 ) ) ;
#4388=CARTESIAN_POINT ( 'NONE',  ( 102.5304832720488832, -102.5304832720499633, 27.50000000000000000 ) ) ;
#4390=VERTEX_POINT ( 'NONE', #6995 ) ;
#4396=CARTESIAN_POINT ( 'NONE',  ( 0.000000000000000000, 0.000000000000000000, 32.50000000000000000 ) ) ;
#4411=DIRECTION ( 'NONE',  ( -0.000000000000000000, -0.000000000000000000, 1.000000000000000000 ) ) ;
#4412=ORIENTED_EDGE ( 'NONE', *, *, #9782, .F. ) ;
#4420=CIRCLE ( 'NONE', #33151, 3.500000000000003109 ) ;
#4422=CYLINDRICAL_SURFACE ( 'NONE', #21353, 25.00000000000000711 ) ;
#4438=DIRECTION ( 'NONE',  ( 0.000000000000000000, 0.000000000000000000, 1.000000000000000000 ) ) ;
#4446=CARTESIAN_POINT ( 'NONE',  ( -145.0000000000000568, 1.518182058997189877E-12, 32.50000000000000000 ) ) ;
#4451=CARTESIAN_POINT ( 'NONE',  ( -86.97117154665588146, 72.12339944410946657, 32.50000000000000711 ) ) ;
#4457=CIRCLE ( 'NONE', #34995, 3.500000000000003109 ) ;
#4458=DIRECTION ( 'NONE',  ( -0.000000000000000000, -0.000000000000000000, -1.000000000000000000 ) ) ;
#4461=VERTEX_POINT ( 'NONE', #5308 ) ;
#4481=ORIENTED_EDGE ( 'NONE', *, *, #12721, .T. ) ;
#4496=DIRECTION ( 'NONE',  ( -0.000000000000000000, -0.000000000000000000, 1.000000000000000000 ) ) ;
#4532=DIRECTION ( 'NONE',  ( -0.000000000000000000, -0.000000000000000000, 1.000000000000000000 ) ) ;
#4570=VERTEX_POINT ( 'NONE', #14636 ) ;
#4579=ORIENTED_EDGE ( 'NONE', *, *, #29895, .F. ) ;
#4583=AXIS2_PLACEMENT_3D ( 'NONE', #25778, #34035, #11500 ) ;
#4599=ORIENTED_EDGE ( 'NONE', *, *, #25860, .T. ) ;
#4648=AXIS2_PLACEMENT_3D ( 'NONE', #18308, #24127, #35406 ) ;
#4649=CARTESIAN_POINT ( 'NONE',  ( -78.83845375417729429, 72.26717041423300714, 32.50000000000000000 ) ) ;
#4650=EDGE_CURVE ( 'NONE', #31750, #8057, #22740, .T. ) ;
#4657=DIRECTION ( 'NONE',  ( 1.000000000000000000, 0.000000000000000000, 0.000000000000000000 ) ) ;
#4659=EDGE_CURVE ( 'NONE', #36154, #31806, #26677, .T. ) ;
#4673=CARTESIAN_POINT ( 'NONE',  ( -98.28784258493107018, -106.7731239591678474, 32.55002500000000509 ) ) ;
#4682=VERTEX_POINT ( 'NONE', #37 ) ;
#4684=VERTEX_POINT ( 'NONE', #2654 ) ;
#4686=DIRECTION ( 'NONE',  ( -0.000000000000000000, -0.000000000000000000, -1.000000000000000000 ) ) ;
#4687=EDGE_LOOP ( 'NONE', ( #14212, #31202 ) ) ;
#4712=DIRECTION ( 'NONE',  ( -0.000000000000000000, -0.000000000000000000, 1.000000000000000000 ) ) ;
#4717=ORIENTED_EDGE ( 'NONE', *, *, #12027, .T. ) ;
#4725=ADVANCED_FACE ( 'NONE', ( #6038 ), #17461, .T. ) ;
#4738=EDGE_CURVE ( 'NONE', #5973, #35680, #6390, .T. ) ;
#4764=EDGE_CURVE ( 'NONE', #3013, #16096, #12738, .T. ) ;
#4773=EDGE_LOOP ( 'NONE', ( #591, #11084, #19226, #3528 ) ) ;
#4789=DIRECTION ( 'NONE',  ( -0.000000000000000000, -0.000000000000000000, -1.000000000000000000 ) ) ;
#4795=DIRECTION ( 'NONE',  ( -1.000000000000000000, 0.000000000000000000, 0.000000000000000000 ) ) ;
#4828=ORIENTED_EDGE ( 'NONE', *, *, #7003, .F. ) ;
#4840=CARTESIAN_POINT ( 'NONE',  ( -106.4311476201816618, 54.27652618157941333, 32.50000000000000000 ) ) ;
#4884=ORIENTED_EDGE ( 'NONE', *, *, #26797, .T. ) ;
#4889=ORIENTED_EDGE ( 'NONE', *, *, #12721, .F. ) ;
#4935=CARTESIAN_POINT ( 'NONE',  ( -107.2724133595221190, -47.49999999999924682, 27.50000000000000000 ) ) ;
#4957=EDGE_CURVE ( 'NONE', #23321, #7276, #8751, .T. ) ;
#4958=DIRECTION ( 'NONE',  ( -1.000000000000000000, 0.000000000000000000, 0.000000000000000000 ) ) ;
#4962=DIRECTION ( 'NONE',  ( 1.000000000000000000, 0.000000000000000000, 0.000000000000000000 ) ) ;
#4963=AXIS2_PLACEMENT_3D ( 'NONE', #16473, #27905, #2785 ) ;
#5002=FACE_OUTER_BOUND ( 'NONE', #35247, .T. ) ;
#5022=CARTESIAN_POINT ( 'NONE',  ( -94.40806000769299544, 12.15049814296761888, 32.50002500000000083 ) ) ;
#5026=CARTESIAN_POINT ( 'NONE',  ( -110.2237710830522559, 101.7384897088162745, 32.50000000000000000 ) ) ;
#5029=EDGE_CURVE ( 'NONE', #13276, #29025, #5168, .T. ) ;
#5042=CARTESIAN_POINT ( 'NONE',  ( 100.6561618467704022, -64.69993787454495759, 32.50000000000000711 ) ) ;
#5043=CARTESIAN_POINT ( 'NONE',  ( -81.11569332658579867, -72.50431249219097651, 32.50000000000000000 ) ) ;
#5045=DIRECTION ( 'NONE',  ( 0.7071067811865489050, 0.7071067811865461294, -0.000000000000000000 ) ) ;
#5049=ORIENTED_EDGE ( 'NONE', *, *, #26843, .T. ) ;
#5059=EDGE_CURVE ( 'NONE', #13060, #10748, #18129, .T. ) ;
#5071=VERTEX_POINT ( 'NONE', #24521 ) ;
#5091=CARTESIAN_POINT ( 'NONE',  ( -111.8061974404900241, -19.22934205794863516, 32.50000000000000000 ) ) ;
#5100=CARTESIAN_POINT ( 'NONE',  ( -102.3447678185619765, -32.57924816083560415, 32.50000000000000711 ) ) ;
#5103=ADVANCED_FACE ( 'NONE', ( #29745 ), #4081, .F. ) ;
#5106=ADVANCED_FACE ( 'NONE', ( #35519 ), #7207, .F. ) ;
#5121=CARTESIAN_POINT ( 'NONE',  ( 98.28784258493033121, 106.7731239591685437, 32.55002500000000509 ) ) ;
#5135=CARTESIAN_POINT ( 'NONE',  ( 12.25360715556858082, 116.9391558507879409, 27.49998799999999477 ) ) ;
#5141=CARTESIAN_POINT ( 'NONE',  ( -70.80619744048887299, 84.18124734178336155, 32.50000000000000000 ) ) ;
#5168=CIRCLE ( 'NONE', #10542, 30.00000000000000000 ) ;
#5174=ORIENTED_EDGE ( 'NONE', *, *, #33991, .F. ) ;
#5178=DIRECTION ( 'NONE',  ( 1.000000000000000000, 0.000000000000000000, 0.000000000000000000 ) ) ;
#5205=EDGE_CURVE ( 'NONE', #30153, #35680, #8773, .T. ) ;
#5225=CARTESIAN_POINT ( 'NONE',  ( 5.999999999999998224, 145.0000000000000568, 32.55002500000000509 ) ) ;
#5248=VECTOR ( 'NONE', #16463, 1000.000000000000000 ) ;
#5253=LINE ( 'NONE', #22306, #16858 ) ;
#5265=CIRCLE ( 'NONE', #19055, 6.000000000000005329 ) ;
#5289=DIRECTION ( 'NONE',  ( 0.000000000000000000, 0.000000000000000000, 1.000000000000000000 ) ) ;
#5295=FACE_OUTER_BOUND ( 'NONE', #32949, .T. ) ;
#5308=CARTESIAN_POINT ( 'NONE',  ( -40.99999999999999289, -103.4105893997321743, 27.50000000000000000 ) ) ;
#5314=ORIENTED_EDGE ( 'NONE', *, *, #33427, .F. ) ;
#5334=CIRCLE ( 'NONE', #13694, 3.500000000000003109 ) ;
#5338=EDGE_CURVE ( 'NONE', #1224, #7201, #2497, .T. ) ;
#5340=EDGE_CURVE ( 'NONE', #2614, #18383, #36798, .T. ) ;
#5356=ORIENTED_EDGE ( 'NONE', *, *, #3035, .T. ) ;
#5367=ORIENTED_EDGE ( 'NONE', *, *, #20817, .T. ) ;
#5373=VERTEX_POINT ( 'NONE', #4935 ) ;
#5375=CARTESIAN_POINT ( 'NONE',  ( 51.68138994340220904, -113.8157894736842053, 32.50000000000000000 ) ) ;
#5381=CARTESIAN_POINT ( 'NONE',  ( 37.50000000000000000, 103.4105893997321743, 32.50000000000000000 ) ) ;
#5384=EDGE_CURVE ( 'NONE', #17212, #23321, #2113, .T. ) ;
#5393=AXIS2_PLACEMENT_3D ( 'NONE', #10598, #28029, #13592 ) ;
#5424=ORIENTED_EDGE ( 'NONE', *, *, #6812, .T. ) ;
#5430=CARTESIAN_POINT ( 'NONE',  ( 106.8157911955970718, -52.30559212667386504, 32.49999999999999289 ) ) ;
#5433=FACE_OUTER_BOUND ( 'NONE', #31445, .T. ) ;
#5457=ORIENTED_EDGE ( 'NONE', *, *, #20207, .F. ) ;
#5466=CARTESIAN_POINT ( 'NONE',  ( 94.55012560584681580, 9.234378588654079678, 27.50000000000000000 ) ) ;
#5480=DIRECTION ( 'NONE',  ( 0.000000000000000000, 0.000000000000000000, 1.000000000000000000 ) ) ;
#5490=CYLINDRICAL_SURFACE ( 'NONE', #26206, 3.500000000000003109 ) ;
#5495=DIRECTION ( 'NONE',  ( 0.000000000000000000, 0.000000000000000000, 1.000000000000000000 ) ) ;
#5498=DIRECTION ( 'NONE',  ( 1.000000000000000000, -1.047444401652940007E-14, 0.000000000000000000 ) ) ;
#5507=DIRECTION ( 'NONE',  ( 0.000000000000000000, 0.000000000000000000, 1.000000000000000000 ) ) ;
#5509=CARTESIAN_POINT ( 'NONE',  ( -77.93343913441745485, -72.12058696850748163, 32.50002500000000083 ) ) ;
#5510=ORIENTED_EDGE ( 'NONE', *, *, #5029, .T. ) ;
#5514=CARTESIAN_POINT ( 'NONE',  ( 139.0000000000000284, -5.056524707326808249E-13, 32.50000000000000000 ) ) ;
#5517=ORIENTED_EDGE ( 'NONE', *, *, #16507, .T. ) ;
#5520=DIRECTION ( 'NONE',  ( 0.000000000000000000, 0.000000000000000000, 1.000000000000000000 ) ) ;
#5526=CARTESIAN_POINT ( 'NONE',  ( 23.27270485391772681, -104.1536085790715305, 32.50000000000000711 ) ) ;
#5543=DIRECTION ( 'NONE',  ( 0.000000000000000000, 0.000000000000000000, 1.000000000000000000 ) ) ;
#5570=CARTESIAN_POINT ( 'NONE',  ( 39.27785635698568711, -86.50000000000001421, 27.50000000000000000 ) ) ;
#5578=CYLINDRICAL_SURFACE ( 'NONE', #31084, 30.00000000000000000 ) ;
#5588=CARTESIAN_POINT ( 'NONE',  ( 6.123233995736731770E-16, -145.0000000000000568, 32.50000000000000000 ) ) ;
#5594=CARTESIAN_POINT ( 'NONE',  ( -107.0735279439396095, -50.67946230268560015, 32.50000000000000711 ) ) ;
#5595=LINE ( 'NONE', #527, #25016 ) ;
#5611=CARTESIAN_POINT ( 'NONE',  ( -37.50000000000000000, 103.4105893997321743, 32.50000000000000000 ) ) ;
#5619=ORIENTED_EDGE ( 'NONE', *, *, #18404, .T. ) ;
#5642=EDGE_CURVE ( 'NONE', #9908, #1442, #16292, .T. ) ;
#5644=DIRECTION ( 'NONE',  ( 1.000000000000000000, 0.000000000000000000, 0.000000000000000000 ) ) ;
#5663=CIRCLE ( 'NONE', #10454, 95.00000000000001421 ) ;
#5664=ORIENTED_EDGE ( 'NONE', *, *, #20191, .T. ) ;
#5670=ORIENTED_EDGE ( 'NONE', *, *, #5921, .T. ) ;
#5695=DIRECTION ( 'NONE',  ( 0.000000000000000000, 0.000000000000000000, 1.000000000000000000 ) ) ;
#5718=CYLINDRICAL_SURFACE ( 'NONE', #6094, 3.500000000000003109 ) ;
#5733=DIRECTION ( 'NONE',  ( 0.000000000000000000, 0.000000000000000000, 1.000000000000000000 ) ) ;
#5760=DIRECTION ( 'NONE',  ( -1.000000000000000000, 0.000000000000000000, 0.000000000000000000 ) ) ;
#5779=AXIS2_PLACEMENT_3D ( 'NONE', #32423, #20803, #23816 ) ;
#5789=EDGE_CURVE ( 'NONE', #16751, #22685, #30440, .T. ) ;
#5792=CARTESIAN_POINT ( 'NONE',  ( 105.2115705174360016, -57.76812138680612918, 32.50000000000000000 ) ) ;
#5795=DIRECTION ( 'NONE',  ( -0.000000000000000000, -0.000000000000000000, 1.000000000000000000 ) ) ;
#5796=ORIENTED_EDGE ( 'NONE', *, *, #21761, .T. ) ;
#5812=CIRCLE ( 'NONE', #15388, 3.499999999999996003 ) ;
#5820=ORIENTED_EDGE ( 'NONE', *, *, #1607, .F. ) ;
#5829=ORIENTED_EDGE ( 'NONE', *, *, #3233, .T. ) ;
#5833=AXIS2_PLACEMENT_3D ( 'NONE', #3487, #26524, #20707 ) ;
#5876=CARTESIAN_POINT ( 'NONE',  ( -107.2724133595211526, 47.50000000000096634, 27.50000000000000000 ) ) ;
#5891=DIRECTION ( 'NONE',  ( 0.000000000000000000, 0.000000000000000000, 1.000000000000000000 ) ) ;
#5902=DIRECTION ( 'NONE',  ( 1.000000000000000000, 0.000000000000000000, 0.000000000000000000 ) ) ;
#5921=EDGE_CURVE ( 'NONE', #28766, #22882, #13010, .T. ) ;
#5927=DIRECTION ( 'NONE',  ( 0.000000000000000000, 0.000000000000000000, 1.000000000000000000 ) ) ;
#5934=ORIENTED_EDGE ( 'NONE', *, *, #29349, .T. ) ;
#5940=ORIENTED_EDGE ( 'NONE', *, *, #14639, .T. ) ;
#5973=VERTEX_POINT ( 'NONE', #6132 ) ;
#5985=ORIENTED_EDGE ( 'NONE', *, *, #7149, .F. ) ;
#6019=DIRECTION ( 'NONE',  ( 1.000000000000000000, 0.000000000000000000, 0.000000000000000000 ) ) ;
#6024=ORIENTED_EDGE ( 'NONE', *, *, #34641, .F. ) ;
#6038=FACE_OUTER_BOUND ( 'NONE', #26405, .T. ) ;
#6042=VERTEX_POINT ( 'NONE', #32942 ) ;
#6047=ORIENTED_EDGE ( 'NONE', *, *, #21822, .F. ) ;
#6052=VERTEX_POINT ( 'NONE', #1617 ) ;
#6056=FACE_OUTER_BOUND ( 'NONE', #32004, .T. ) ;
#6062=CARTESIAN_POINT ( 'NONE',  ( -72.72667006428976322, 101.6652913307188868, 32.50002500000000083 ) ) ;
#6065=ADVANCED_FACE ( 'NONE', ( #35575 ), #15509, .T. ) ;
#6075=DIRECTION ( 'NONE',  ( 0.000000000000000000, 0.000000000000000000, 1.000000000000000000 ) ) ;
#6091=ORIENTED_EDGE ( 'NONE', *, *, #3763, .T. ) ;
#6094=AXIS2_PLACEMENT_3D ( 'NONE', #28589, #3468, #2923 ) ;
#6103=ORIENTED_EDGE ( 'NONE', *, *, #18304, .F. ) ;
#6107=ORIENTED_EDGE ( 'NONE', *, *, #8478, .F. ) ;
#6122=EDGE_CURVE ( 'NONE', #22882, #32886, #7642, .T. ) ;
#6132=CARTESIAN_POINT ( 'NONE',  ( -104.8061974404896262, 19.22934205795090534, 27.50000000000000000 ) ) ;
#6168=EDGE_LOOP ( 'NONE', ( #11472, #8715 ) ) ;
#6176=ADVANCED_FACE ( 'NONE', ( #36508 ), #28399, .F. ) ;
#6178=CARTESIAN_POINT ( 'NONE',  ( 84.91058168688746832, 72.42202624339670081, 32.50000000000000711 ) ) ;
#6185=ORIENTED_EDGE ( 'NONE', *, *, #28124, .F. ) ;
#6195=DIRECTION ( 'NONE',  ( 0.000000000000000000, 0.000000000000000000, 1.000000000000000000 ) ) ;
#6196=ORIENTED_EDGE ( 'NONE', *, *, #34736, .F. ) ;
#6200=FACE_BOUND ( 'NONE', #23600, .T. ) ;
#6205=ORIENTED_EDGE ( 'NONE', *, *, #33798, .T. ) ;
#6215=CARTESIAN_POINT ( 'NONE',  ( -77.93337901593650940, -72.12093275448718543, 32.50001250000000397 ) ) ;
#6220=EDGE_CURVE ( 'NONE', #24561, #18446, #36310, .T. ) ;
#6228=VERTEX_POINT ( 'NONE', #34061 ) ;
#6237=ORIENTED_EDGE ( 'NONE', *, *, #36344, .T. ) ;
#6254=VECTOR ( 'NONE', #23830, 1000.000000000000000 ) ;
#6260=EDGE_CURVE ( 'NONE', #35608, #35112, #7054, .T. ) ;
#6263=CIRCLE ( 'NONE', #8647, 95.00000000000001421 ) ;
#6277=EDGE_LOOP ( 'NONE', ( #17235, #4884, #33763, #23087 ) ) ;
#6283=CIRCLE ( 'NONE', #8692, 150.0000000000000284 ) ;
#6303=EDGE_CURVE ( 'NONE', #6715, #4682, #12435, .T. ) ;
#6315=ORIENTED_EDGE ( 'NONE', *, *, #25901, .F. ) ;
#6326=LINE ( 'NONE', #11411, #26204 ) ;
#6328=VECTOR ( 'NONE', #24192, 1000.000000000000000 ) ;
#6348=CARTESIAN_POINT ( 'NONE',  ( -101.4252628994512833, -31.43180897937256191, 32.50001250000000397 ) ) ;
#6359=ORIENTED_EDGE ( 'NONE', *, *, #14558, .F. ) ;
#6361=EDGE_CURVE ( 'NONE', #2049, #40, #31930, .T. ) ;
#6367=PLANE ( 'NONE',  #35116 ) ;
#6389=CARTESIAN_POINT ( 'NONE',  ( 0.000000000000000000, 0.000000000000000000, 32.50000000000000000 ) ) ;
#6390=LINE ( 'NONE', #15759, #6328 ) ;
#6396=SHAPE_REPRESENTATION ( 'mounting backplate', ( #21385 ), #25533 ) ;
#6418=LINE ( 'NONE', #36217, #20088 ) ;
#6430=EDGE_CURVE ( 'NONE', #8770, #23345, #5265, .T. ) ;
#6435=EDGE_CURVE ( 'NONE', #22752, #17730, #22044, .T. ) ;
#6442=DIRECTION ( 'NONE',  ( 0.000000000000000000, 0.000000000000000000, 1.000000000000000000 ) ) ;
#6445=CARTESIAN_POINT ( 'NONE',  ( 0.000000000000000000, 0.000000000000000000, 27.50000000000000000 ) ) ;
#6450=EDGE_CURVE ( 'NONE', #9234, #15626, #28615, .T. ) ;
#6454=CARTESIAN_POINT ( 'NONE',  ( -145.0000000000001137, -5.999999999998481215, 32.50000000000000000 ) ) ;
#6460=CIRCLE ( 'NONE', #2884, 30.00000000000000000 ) ;
#6469=VECTOR ( 'NONE', #17471, 1000.000000000000000 ) ;
#6511=DIRECTION ( 'NONE',  ( 1.000000000000000000, 0.000000000000000000, 0.000000000000000000 ) ) ;
#6513=EDGE_LOOP ( 'NONE', ( #23879, #27884, #7382, #28237 ) ) ;
#6524=CARTESIAN_POINT ( 'NONE',  ( 67.30619744048945563, -84.18124734178287838, 27.50000000000000000 ) ) ;
#6527=DIRECTION ( 'NONE',  ( 0.000000000000000000, 0.000000000000000000, 1.000000000000000000 ) ) ;
#6528=EDGE_CURVE ( 'NONE', #32462, #16311, #6460, .T. ) ;
#6542=ADVANCED_FACE ( 'NONE', ( #21255 ), #1768, .F. ) ;
#6545=ORIENTED_EDGE ( 'NONE', *, *, #6361, .F. ) ;
#6563=PLANE ( 'NONE',  #23970 ) ;
#6583=EDGE_CURVE ( 'NONE', #3455, #15010, #7385, .T. ) ;
#6585=VECTOR ( 'NONE', #4712, 1000.000000000000000 ) ;
#6586=FACE_BOUND ( 'NONE', #11584, .T. ) ;
#6587=CARTESIAN_POINT ( 'NONE',  ( -6.000000000000000000, 145.0000000000000568, 32.55002500000000509 ) ) ;
#6609=DIRECTION ( 'NONE',  ( 0.000000000000000000, 0.000000000000000000, 1.000000000000000000 ) ) ;
#6612=EDGE_CURVE ( 'NONE', #30149, #20872, #11956, .T. ) ;
#6632=CARTESIAN_POINT ( 'NONE',  ( -2.577278915392902991, -120.0000464694457776, 32.50000000000000711 ) ) ;
#6652=DIRECTION ( 'NONE',  ( 0.000000000000000000, 0.000000000000000000, 1.000000000000000000 ) ) ;
#6653=CARTESIAN_POINT ( 'NONE',  ( -70.80619744049063513, -84.18124734178186941, 32.50000000000000000 ) ) ;
#6661=EDGE_CURVE ( 'NONE', #23345, #2049, #35334, .T. ) ;
#6672=EDGE_CURVE ( 'NONE', #20316, #8483, #12548, .T. ) ;
#6675=CARTESIAN_POINT ( 'NONE',  ( -108.3061974404896262, 19.22934205795090534, 32.50000000000000000 ) ) ;
#6678=LINE ( 'NONE', #26730, #35355 ) ;
#6681=DIRECTION ( 'NONE',  ( -0.000000000000000000, -0.000000000000000000, 1.000000000000000000 ) ) ;
#6705=DIRECTION ( 'NONE',  ( 1.000000000000000000, 0.000000000000000000, 0.000000000000000000 ) ) ;
#6712=ORIENTED_EDGE ( 'NONE', *, *, #12096, .F. ) ;
#6715=VERTEX_POINT ( 'NONE', #36592 ) ;
#6728=EDGE_CURVE ( 'NONE', #8890, #12147, #21559, .T. ) ;
#6732=DIRECTION ( 'NONE',  ( 1.000000000000000000, 0.000000000000000000, 0.000000000000000000 ) ) ;
#6735=CARTESIAN_POINT ( 'NONE',  ( 101.8359879928019893, 31.92197653850545436, 32.50000000000000000 ) ) ;
#6736=LINE ( 'NONE', #18169, #2212 ) ;
#6739=CIRCLE ( 'NONE', #33683, 3.499999999999996003 ) ;
#6752=AXIS2_PLACEMENT_3D ( 'NONE', #2133, #16581, #22211 ) ;
#6755=CARTESIAN_POINT ( 'NONE',  ( -67.30619744048885877, 84.18124734178336155, 32.50000000000000000 ) ) ;
#6774=PLANE ( 'NONE',  #31472 ) ;
#6794=ORIENTED_EDGE ( 'NONE', *, *, #30284, .F. ) ;
#6812=EDGE_CURVE ( 'NONE', #6228, #19610, #7900, .T. ) ;
#6846=CYLINDRICAL_SURFACE ( 'NONE', #19762, 30.00000000000001421 ) ;
#6851=DIRECTION ( 'NONE',  ( -1.000000000000000000, 0.000000000000000000, 0.000000000000000000 ) ) ;
#6872=EDGE_LOOP ( 'NONE', ( #6196, #10026 ) ) ;
#6920=DIRECTION ( 'NONE',  ( 0.000000000000000000, 0.000000000000000000, 1.000000000000000000 ) ) ;
#6924=CARTESIAN_POINT ( 'NONE',  ( 106.8646861230860878, 42.81779240327628600, 32.50000000000000000 ) ) ;
#6929=VECTOR ( 'NONE', #18494, 1000.000000000000000 ) ;
#6959=ORIENTED_EDGE ( 'NONE', *, *, #34953, .F. ) ;
#6961=VECTOR ( 'NONE', #3089, 1000.000000000000000 ) ;
#6992=ADVANCED_FACE ( 'NONE', ( #12544 ), #21167, .F. ) ;
#6995=CARTESIAN_POINT ( 'NONE',  ( -5.999999999999985789, -149.8799519615616305, 32.50000000000000000 ) ) ;
#6997=PRODUCT_DEFINITION ( 'UNKNOWN', '', #12966, #2443 ) ;
#7003=EDGE_CURVE ( 'NONE', #1358, #15010, #15735, .T. ) ;
#7022=DIRECTION ( 'NONE',  ( 0.000000000000000000, 0.000000000000000000, 1.000000000000000000 ) ) ;
#7042=CARTESIAN_POINT ( 'NONE',  ( 98.28784258493033121, 106.7731239591685437, 32.50000000000000000 ) ) ;
#7054=CIRCLE ( 'NONE', #29818, 3.499999999999996003 ) ;
#7059=CARTESIAN_POINT ( 'NONE',  ( 101.7384897088143560, -110.2237710830540180, 32.50000000000000000 ) ) ;
#7067=CARTESIAN_POINT ( 'NONE',  ( -98.28784258493107018, -106.7731239591678474, 32.50000000000000000 ) ) ;
#7099=VECTOR ( 'NONE', #5498, 1000.000000000000000 ) ;
#7100=EDGE_CURVE ( 'NONE', #17212, #20372, #4223, .T. ) ;
#7116=ADVANCED_FACE ( 'NONE', ( #29595 ), #6563, .F. ) ;
#7117=VECTOR ( 'NONE', #10301, 1000.000000000000000 ) ;
#7130=AXIS2_PLACEMENT_3D ( 'NONE', #3770, #7472, #34914 ) ;
#7133=CARTESIAN_POINT ( 'NONE',  ( 104.0323809747665109, -35.06837973811266096, 32.50000000000000000 ) ) ;
#7138=ORIENTED_EDGE ( 'NONE', *, *, #28796, .F. ) ;
#7143=CARTESIAN_POINT ( 'NONE',  ( 37.50000000000000000, -103.4105893997321743, 27.50000000000000000 ) ) ;
#7149=EDGE_CURVE ( 'NONE', #9158, #10452, #28168, .T. ) ;
#7163=ORIENTED_EDGE ( 'NONE', *, *, #33023, .T. ) ;
#7168=DIRECTION ( 'NONE',  ( 1.000000000000000000, 0.000000000000000000, 0.000000000000000000 ) ) ;
#7173=ORIENTED_EDGE ( 'NONE', *, *, #18340, .T. ) ;
#7174=DIRECTION ( 'NONE',  ( -0.000000000000000000, 0.000000000000000000, -1.000000000000000000 ) ) ;
#7175=FACE_OUTER_BOUND ( 'NONE', #25270, .T. ) ;
#7201=VERTEX_POINT ( 'NONE', #36719 ) ;
#7206=CARTESIAN_POINT ( 'NONE',  ( -6.000000000000000000, 149.8799519615616305, 27.50000000000000000 ) ) ;
#7207=CYLINDRICAL_SURFACE ( 'NONE', #3396, 24.99999999999999289 ) ;
#7212=DIRECTION ( 'NONE',  ( 0.000000000000000000, 0.000000000000000000, 1.000000000000000000 ) ) ;
#7216=DIRECTION ( 'NONE',  ( -0.000000000000000000, -0.000000000000000000, -1.000000000000000000 ) ) ;
#7218=CARTESIAN_POINT ( 'NONE',  ( 70.80619744048946984, -84.18124734178287838, 27.50000000000000000 ) ) ;
#7230=VERTEX_POINT ( 'NONE', #16299 ) ;
#7234=VERTEX_POINT ( 'NONE', #2229 ) ;
#7237=EDGE_LOOP ( 'NONE', ( #22423, #7862, #12608, #30672 ) ) ;
#7268=DIRECTION ( 'NONE',  ( -0.000000000000000000, -0.000000000000000000, -1.000000000000000000 ) ) ;
#7271=CARTESIAN_POINT ( 'NONE',  ( -78.38321060269107932, 72.20005542350995142, 32.50000000000000000 ) ) ;
#7276=VERTEX_POINT ( 'NONE', #3829 ) ;
#7278=CARTESIAN_POINT ( 'NONE',  ( 34.00000000000000000, -103.4105893997321743, 27.50000000000000000 ) ) ;
#7295=ORIENTED_EDGE ( 'NONE', *, *, #25930, .T. ) ;
#7309=ADVANCED_FACE ( 'NONE', ( #20913 ), #23721, .F. ) ;
#7316=DIRECTION ( 'NONE',  ( 0.000000000000000000, -0.000000000000000000, -1.000000000000000000 ) ) ;
#7330=( NAMED_UNIT ( * ) PLANE_ANGLE_UNIT ( ) SI_UNIT ( $, .RADIAN. ) );
#7350=AXIS2_PLACEMENT_3D ( 'NONE', #28499, #2833, #23057 ) ;
#7357=CARTESIAN_POINT ( 'NONE',  ( -108.3061974404896262, 19.22934205795090534, 27.50000000000000000 ) ) ;
#7359=CARTESIAN_POINT ( 'NONE',  ( 55.27226924886075921, -77.26562141134597539, 27.50000000000000000 ) ) ;
#7370=ORIENTED_EDGE ( 'NONE', *, *, #6220, .F. ) ;
#7375=ORIENTED_EDGE ( 'NONE', *, *, #33593, .F. ) ;
#7382=ORIENTED_EDGE ( 'NONE', *, *, #8737, .T. ) ;
#7385=LINE ( 'NONE', #33253, #22773 ) ;
#7412=LINE ( 'NONE', #13786, #35089 ) ;
#7414=FACE_BOUND ( 'NONE', #17685, .T. ) ;
#7459=EDGE_LOOP ( 'NONE', ( #29243, #15773 ) ) ;
#7472=DIRECTION ( 'NONE',  ( -0.000000000000000000, -0.000000000000000000, 1.000000000000000000 ) ) ;
#7521=VERTEX_POINT ( 'NONE', #10219 ) ;
#7530=ADVANCED_FACE ( 'NONE', ( #29697 ), #21647, .F. ) ;
#7531=DIRECTION ( 'NONE',  ( 1.000000000000000000, 0.000000000000000000, 0.000000000000000000 ) ) ;
#7532=VERTEX_POINT ( 'NONE', #32902 ) ;
#7564=CARTESIAN_POINT ( 'NONE',  ( 101.4249800177813086, -31.43204461043964315, 32.50002500000000083 ) ) ;
#7584=CARTESIAN_POINT ( 'NONE',  ( -5.999999999999985789, -149.8799519615616305, 32.55002500000000509 ) ) ;
#7587=EDGE_CURVE ( 'NONE', #31164, #24047, #27547, .T. ) ;
#7607=DIRECTION ( 'NONE',  ( 1.000000000000000000, 0.000000000000000000, 0.000000000000000000 ) ) ;
#7610=EDGE_CURVE ( 'NONE', #25010, #4390, #25157, .T. ) ;
#7614=CARTESIAN_POINT ( 'NONE',  ( 111.8061974404898962, 19.22934205794938478, 27.50000000000000000 ) ) ;
#7641=CARTESIAN_POINT ( 'NONE',  ( -70.80619744048887299, 84.18124734178336155, 27.50000000000000000 ) ) ;
#7642=CIRCLE ( 'NONE', #4648, 95.00000000000001421 ) ;
#7650=ORIENTED_EDGE ( 'NONE', *, *, #5642, .T. ) ;
#7671=ORIENTED_EDGE ( 'NONE', *, *, #5789, .T. ) ;
#7705=ORIENTED_EDGE ( 'NONE', *, *, #9539, .F. ) ;
#7739=DIRECTION ( 'NONE',  ( 1.000000000000000000, 0.000000000000000000, 0.000000000000000000 ) ) ;
#7748=AXIS2_PLACEMENT_3D ( 'NONE', #9825, #21260, #1388 ) ;
#7780=AXIS2_PLACEMENT_3D ( 'NONE', #15968, #9962, #7168 ) ;
#7794=FACE_BOUND ( 'NONE', #9244, .T. ) ;
#7814=DIRECTION ( 'NONE',  ( -0.000000000000000000, -0.000000000000000000, 1.000000000000000000 ) ) ;
#7823=ORIENTED_EDGE ( 'NONE', *, *, #8229, .F. ) ;
#7838=CARTESIAN_POINT ( 'NONE',  ( -107.2750611683612192, 48.40478642138986487, 32.50000000000000711 ) ) ;
#7841=FACE_OUTER_BOUND ( 'NONE', #10741, .T. ) ;
#7862=ORIENTED_EDGE ( 'NONE', *, *, #5340, .T. ) ;
#7874=CARTESIAN_POINT ( 'NONE',  ( 105.1746053637160117, -37.32370766915258287, 32.49999999999999289 ) ) ;
#7881=SURFACE_SIDE_STYLE ('',( #33173 ) ) ;
#7900=LINE ( 'NONE', #2070, #18571 ) ;
#7905=CARTESIAN_POINT ( 'NONE',  ( 0.000000000000000000, -95.00000000000001421, 27.50000000000000000 ) ) ;
#7907=EDGE_CURVE ( 'NONE', #7234, #13265, #26977, .T. ) ;
#7916=DIRECTION ( 'NONE',  ( 1.000000000000000000, 0.000000000000000000, 0.000000000000000000 ) ) ;
#7919=ORIENTED_EDGE ( 'NONE', *, *, #29826, .F. ) ;
#7920=ORIENTED_EDGE ( 'NONE', *, *, #14566, .F. ) ;
#7926=EDGE_LOOP ( 'NONE', ( #20969, #33170, #11499, #24166 ) ) ;
#7938=ORIENTED_EDGE ( 'NONE', *, *, #6430, .T. ) ;
#7947=ADVANCED_FACE ( 'NONE', ( #7175 ), #976, .F. ) ;
#7953=ORIENTED_EDGE ( 'NONE', *, *, #9539, .T. ) ;
#7983=CARTESIAN_POINT ( 'NONE',  ( -108.3061974404896262, 19.22934205795090534, 32.50000000000000000 ) ) ;
#7996=ORIENTED_EDGE ( 'NONE', *, *, #27050, .F. ) ;
#8000=VECTOR ( 'NONE', #9020, 1000.000000000000000 ) ;
#8024=CARTESIAN_POINT ( 'NONE',  ( 55.27226924886128501, 77.26562141134559170, 32.50000000000000000 ) ) ;
#8039=DIRECTION ( 'NONE',  ( 1.000000000000000000, 0.000000000000000000, 0.000000000000000000 ) ) ;
#8047=DIRECTION ( 'NONE',  ( -0.000000000000000000, -0.000000000000000000, -1.000000000000000000 ) ) ;
#8048=DIRECTION ( 'NONE',  ( -0.000000000000000000, -0.000000000000000000, -1.000000000000000000 ) ) ;
#8053=UNCERTAINTY_MEASURE_WITH_UNIT (LENGTH_MEASURE( 1.000000000000000082E-05 ), #16328, 'distance_accuracy_value', 'NONE');
#8057=VERTEX_POINT ( 'NONE', #16894 ) ;
#8087=DIRECTION ( 'NONE',  ( -0.000000000000000000, -0.000000000000000000, 1.000000000000000000 ) ) ;
#8115=VERTEX_POINT ( 'NONE', #14273 ) ;
#8126=DIRECTION ( 'NONE',  ( -0.000000000000000000, -0.000000000000000000, -1.000000000000000000 ) ) ;
#8139=CIRCLE ( 'NONE', #26705, 3.500000000000003109 ) ;
#8146=LINE ( 'NONE', #30470, #23842 ) ;
#8149=FACE_OUTER_BOUND ( 'NONE', #20050, .T. ) ;
#8179=ORIENTED_EDGE ( 'NONE', *, *, #14347, .T. ) ;
#8186=ORIENTED_EDGE ( 'NONE', *, *, #6122, .F. ) ;
#8196=AXIS2_PLACEMENT_3D ( 'NONE', #11365, #16984, #10817 ) ;
#8204=ORIENTED_EDGE ( 'NONE', *, *, #21128, .T. ) ;
#8229=EDGE_CURVE ( 'NONE', #16622, #27555, #25882, .T. ) ;
#8239=CARTESIAN_POINT ( 'NONE',  ( -96.90588911714331743, -67.77518747868774085, 32.49999999999998579 ) ) ;
#8259=AXIS2_PLACEMENT_3D ( 'NONE', #20161, #17521, #18081 ) ;
#8267=ORIENTED_EDGE ( 'NONE', *, *, #15163, .T. ) ;
#8280=CARTESIAN_POINT ( 'NONE',  ( 0.000000000000000000, 0.000000000000000000, 32.50000000000000000 ) ) ;
#8282=ADVANCED_FACE ( 'NONE', ( #23820 ), #18744, .T. ) ;
#8347=CARTESIAN_POINT ( 'NONE',  ( -111.8061974404896262, 19.22934205795090534, 27.50000000000000000 ) ) ;
#8352=CARTESIAN_POINT ( 'NONE',  ( 20.26402367686958428, -109.7457339126789151, 32.50000000000000711 ) ) ;
#8379=CYLINDRICAL_SURFACE ( 'NONE', #20151, 3.500000000000003109 ) ;
#8416=VECTOR ( 'NONE', #20262, 1000.000000000000000 ) ;
#8424=CARTESIAN_POINT ( 'NONE',  ( -77.93337901593650940, -72.12093275448718543, 32.50001250000000397 ) ) ;
#8426=CARTESIAN_POINT ( 'NONE',  ( -6.000000000000000000, 145.0000000000000568, 27.50000000000000000 ) ) ;
#8437=ORIENTED_EDGE ( 'NONE', *, *, #34019, .T. ) ;
#8456=LINE ( 'NONE', #13886, #25529 ) ;
#8462=CARTESIAN_POINT ( 'NONE',  ( -106.7731239591675205, 98.28784258493142545, 27.50000000000000000 ) ) ;
#8470=CARTESIAN_POINT ( 'NONE',  ( -70.80619744048887299, 84.18124734178336155, 27.50000000000000000 ) ) ;
#8475=CARTESIAN_POINT ( 'NONE',  ( -145.0000000000000000, 6.000000000001517009, 32.55002500000000509 ) ) ;
#8478=EDGE_CURVE ( 'NONE', #28544, #3789, #19817, .T. ) ;
#8483=VERTEX_POINT ( 'NONE', #3532 ) ;
#8501=CARTESIAN_POINT ( 'NONE',  ( -22.62085422049824501, 105.9441492178757898, 27.49998800000000543 ) ) ;
#8512=CARTESIAN_POINT ( 'NONE',  ( -51.68138994340220904, -113.8157894736842053, 32.50000000000000000 ) ) ;
#8534=DIRECTION ( 'NONE',  ( 1.000000000000000000, 0.000000000000000000, 0.000000000000000000 ) ) ;
#8568=FACE_OUTER_BOUND ( 'NONE', #7237, .T. ) ;
#8588=CARTESIAN_POINT ( 'NONE',  ( 106.1304126751635835, -55.40976756914862023, 32.50000000000002132 ) ) ;
#8589=DIRECTION ( 'NONE',  ( -0.000000000000000000, 1.000000000000000000, 0.000000000000000000 ) ) ;
#8607=CARTESIAN_POINT ( 'NONE',  ( 102.5304832720488832, -102.5304832720499633, 27.50000000000000000 ) ) ;
#8613=EDGE_CURVE ( 'NONE', #37066, #31750, #34807, .T. ) ;
#8647=AXIS2_PLACEMENT_3D ( 'NONE', #27336, #1100, #18151 ) ;
#8648=DIRECTION ( 'NONE',  ( 0.000000000000000000, 0.000000000000000000, 1.000000000000000000 ) ) ;
#8665=VERTEX_POINT ( 'NONE', #4270 ) ;
#8674=VECTOR ( 'NONE', #22630, 1000.000000000000000 ) ;
#8678=VERTEX_POINT ( 'NONE', #6524 ) ;
#8692=AXIS2_PLACEMENT_3D ( 'NONE', #13130, #33574, #12729 ) ;
#8693=FACE_OUTER_BOUND ( 'NONE', #27094, .T. ) ;
#8697=ORIENTED_EDGE ( 'NONE', *, *, #1490, .T. ) ;
#8708=DIRECTION ( 'NONE',  ( -1.000000000000000000, 0.000000000000000000, 0.000000000000000000 ) ) ;
#8715=ORIENTED_EDGE ( 'NONE', *, *, #8930, .F. ) ;
#8717=DIRECTION ( 'NONE',  ( 1.000000000000000000, 0.000000000000000000, 0.000000000000000000 ) ) ;
#8726=EDGE_CURVE ( 'NONE', #27343, #27468, #12290, .T. ) ;
#8732=ORIENTED_EDGE ( 'NONE', *, *, #24447, .T. ) ;
#8734=DIRECTION ( 'NONE',  ( -0.7071067811865561215, -0.7071067811865389130, 0.000000000000000000 ) ) ;
#8737=EDGE_CURVE ( 'NONE', #22752, #24628, #25084, .T. ) ;
#8748=EDGE_LOOP ( 'NONE', ( #21671, #11461, #7163, #20905 ) ) ;
#8751=CIRCLE ( 'NONE', #9949, 150.0000000000000284 ) ;
#8759=DIRECTION ( 'NONE',  ( -0.000000000000000000, -0.000000000000000000, 1.000000000000000000 ) ) ;
#8761=CARTESIAN_POINT ( 'NONE',  ( 72.72667006429044534, -101.6652913307183610, 32.50002500000000083 ) ) ;
#8770=VERTEX_POINT ( 'NONE', #36131 ) ;
#8773=CIRCLE ( 'NONE', #9354, 3.500000000000003109 ) ;
#8779=FACE_OUTER_BOUND ( 'NONE', #23492, .T. ) ;
#8790=VECTOR ( 'NONE', #13881, 1000.000000000000000 ) ;
#8798=CIRCLE ( 'NONE', #25015, 30.00000000000000000 ) ;
#8804=ORIENTED_EDGE ( 'NONE', *, *, #22911, .T. ) ;
#8807=EDGE_CURVE ( 'NONE', #6042, #33391, #2738, .T. ) ;
#8820=CARTESIAN_POINT ( 'NONE',  ( 4.242640687119251908, -4.242640687119325626, 27.50000000000000000 ) ) ;
#8849=DIRECTION ( 'NONE',  ( 1.000000000000000000, 0.000000000000000000, 0.000000000000000000 ) ) ;
#8863=VECTOR ( 'NONE', #34414, 1000.000000000000000 ) ;
#8870=DIRECTION ( 'NONE',  ( -1.000000000000000000, 0.000000000000000000, 0.000000000000000000 ) ) ;
#8883=CYLINDRICAL_SURFACE ( 'NONE', #32167, 30.00000000000001421 ) ;
#8888=ORIENTED_EDGE ( 'NONE', *, *, #4738, .T. ) ;
#8889=CARTESIAN_POINT ( 'NONE',  ( -19.04446855847336195, -111.2114855601511607, 32.50000000000000711 ) ) ;
#8890=VERTEX_POINT ( 'NONE', #1992 ) ;
#8896=CARTESIAN_POINT ( 'NONE',  ( 0.000000000000000000, 0.000000000000000000, 0.000000000000000000 ) ) ;
#8908=DIRECTION ( 'NONE',  ( 1.000000000000000000, 0.000000000000000000, 0.000000000000000000 ) ) ;
#8911=CARTESIAN_POINT ( 'NONE',  ( 102.5304832720488832, -102.5304832720499633, 32.50000000000000000 ) ) ;
#8930=EDGE_CURVE ( 'NONE', #22685, #16751, #34462, .T. ) ;
#8953=DIRECTION ( 'NONE',  ( -0.000000000000000000, -0.000000000000000000, -1.000000000000000000 ) ) ;
#8957=EDGE_CURVE ( 'NONE', #22752, #3013, #14466, .T. ) ;
#8962=ORIENTED_EDGE ( 'NONE', *, *, #34641, .T. ) ;
#8970=DIRECTION ( 'NONE',  ( -0.000000000000000000, -0.000000000000000000, -1.000000000000000000 ) ) ;
#8978=DIRECTION ( 'NONE',  ( 0.000000000000000000, -0.000000000000000000, -1.000000000000000000 ) ) ;
#8980=DIRECTION ( 'NONE',  ( 1.000000000000000000, 0.000000000000000000, 0.000000000000000000 ) ) ;
#9005=CARTESIAN_POINT ( 'NONE',  ( 108.3061974404897825, -19.22934205795014151, 27.50000000000000000 ) ) ;
#9006=DIRECTION ( 'NONE',  ( 1.000000000000000000, 0.000000000000000000, 0.000000000000000000 ) ) ;
#9020=DIRECTION ( 'NONE',  ( -0.000000000000000000, -0.000000000000000000, -1.000000000000000000 ) ) ;
#9027=ORIENTED_EDGE ( 'NONE', *, *, #22, .F. ) ;
#9040=AXIS2_PLACEMENT_3D ( 'NONE', #27363, #26993, #18575 ) ;
#9048=CARTESIAN_POINT ( 'NONE',  ( -82.27241335952211898, -47.49999999999924682, 32.50002500000000083 ) ) ;
#9053=EDGE_LOOP ( 'NONE', ( #6959, #36530, #27729, #13430 ) ) ;
#9071=DIRECTION ( 'NONE',  ( 1.000000000000000000, 0.000000000000000000, 0.000000000000000000 ) ) ;
#9129=VERTEX_POINT ( 'NONE', #29964 ) ;
#9144=ORIENTED_EDGE ( 'NONE', *, *, #8807, .T. ) ;
#9154=CARTESIAN_POINT ( 'NONE',  ( 39.27785635698568711, -86.50000000000001421, 32.50000000000000000 ) ) ;
#9155=ORIENTED_EDGE ( 'NONE', *, *, #35306, .T. ) ;
#9158=VERTEX_POINT ( 'NONE', #10274 ) ;
#9168=CARTESIAN_POINT ( 'NONE',  ( 80.47882414735005341, 72.44490339922796807, 32.49999999999998579 ) ) ;
#9182=ORIENTED_EDGE ( 'NONE', *, *, #10544, .F. ) ;
#9197=ORIENTED_EDGE ( 'NONE', *, *, #13181, .T. ) ;
#9200=EDGE_LOOP ( 'NONE', ( #16780, #27396, #29159, #20574 ) ) ;
#9217=DIRECTION ( 'NONE',  ( -1.000000000000000000, 0.000000000000000000, 0.000000000000000000 ) ) ;
#9234=VERTEX_POINT ( 'NONE', #12835 ) ;
#9242=EDGE_LOOP ( 'NONE', ( #26798, #19086, #16947, #27586 ) ) ;
#9243=CARTESIAN_POINT ( 'NONE',  ( 101.7384897088143560, -110.2237710830540180, 32.55002500000000509 ) ) ;
#9244=EDGE_LOOP ( 'NONE', ( #31173, #21139 ) ) ;
#9300=AXIS2_PLACEMENT_3D ( 'NONE', #11376, #22634, #19823 ) ;
#9324=CARTESIAN_POINT ( 'NONE',  ( -67.30619744049063513, -84.18124734178186941, 32.50000000000000000 ) ) ;
#9335=AXIS2_PLACEMENT_3D ( 'NONE', #9487, #15097, #26526 ) ;
#9354=AXIS2_PLACEMENT_3D ( 'NONE', #32496, #16012, #12436 ) ;
#9366=CARTESIAN_POINT ( 'NONE',  ( 40.99999999999999289, -103.4105893997321743, 32.50000000000000000 ) ) ;
#9373=ORIENTED_EDGE ( 'NONE', *, *, #19394, .T. ) ;
#9377=ORIENTED_EDGE ( 'NONE', *, *, #17465, .F. ) ;
#9411=SURFACE_STYLE_FILL_AREA ( #28479 ) ;
#9430=AXIS2_PLACEMENT_3D ( 'NONE', #24871, #25246, #36674 ) ;
#9433=EDGE_LOOP ( 'NONE', ( #492, #13691, #35973, #6794 ) ) ;
#9455=DIRECTION ( 'NONE',  ( -0.000000000000000000, -0.000000000000000000, -1.000000000000000000 ) ) ;
#9460=EDGE_CURVE ( 'NONE', #20372, #7276, #32315, .T. ) ;
#9472=AXIS2_PLACEMENT_3D ( 'NONE', #26918, #32153, #1233 ) ;
#9477=CIRCLE ( 'NONE', #17837, 95.00000000000001421 ) ;
#9487=CARTESIAN_POINT ( 'NONE',  ( 108.3061974404898820, 19.22934205794938478, 27.50000000000000000 ) ) ;
#9497=ORIENTED_EDGE ( 'NONE', *, *, #30847, .T. ) ;
#9512=EDGE_LOOP ( 'NONE', ( #17565, #25951, #8888, #13741 ) ) ;
#9524=DIRECTION ( 'NONE',  ( 0.000000000000000000, 0.000000000000000000, 1.000000000000000000 ) ) ;
#9528=VECTOR ( 'NONE', #18942, 1000.000000000000000 ) ;
#9531=ORIENTED_EDGE ( 'NONE', *, *, #26797, .F. ) ;
#9539=EDGE_CURVE ( 'NONE', #10452, #23651, #29316, .T. ) ;
#9563=CARTESIAN_POINT ( 'NONE',  ( 101.0514726702494386, 64.20674970622599176, 32.50000000000001421 ) ) ;
#9580=DIRECTION ( 'NONE',  ( -0.000000000000000000, -0.000000000000000000, 1.000000000000000000 ) ) ;
#9581=CARTESIAN_POINT ( 'NONE',  ( 34.00000000000000000, 103.4105893997321743, 27.50000000000000000 ) ) ;
#9606=CIRCLE ( 'NONE', #27878, 3.500000000000003109 ) ;
#9609=DIRECTION ( 'NONE',  ( -0.7071067811865411334, 0.7071067811865539010, 0.000000000000000000 ) ) ;
#9616=ORIENTED_EDGE ( 'NONE', *, *, #36925, .T. ) ;
#9622=ADVANCED_FACE ( 'NONE', ( #1924 ), #1196, .F. ) ;
#9633=ORIENTED_EDGE ( 'NONE', *, *, #22923, .T. ) ;
#9636=ORIENTED_EDGE ( 'NONE', *, *, #21790, .T. ) ;
#9663=CARTESIAN_POINT ( 'NONE',  ( -108.3061974404900241, -19.22934205794863516, 32.50000000000000000 ) ) ;
#9671=EDGE_CURVE ( 'NONE', #12740, #3455, #13185, .T. ) ;
#9689=CARTESIAN_POINT ( 'NONE',  ( 108.3061974404897825, -19.22934205795014151, 27.50000000000000000 ) ) ;
#9696=CARTESIAN_POINT ( 'NONE',  ( 55.27226924886128501, 77.26562141134559170, 27.50000000000000000 ) ) ;
#9713=DIRECTION ( 'NONE',  ( 1.000000000000000000, -1.047444401652940007E-14, 0.000000000000000000 ) ) ;
#9734=CARTESIAN_POINT ( 'NONE',  ( 86.78953283892636250, 72.09873182956143012, 32.50000000000000000 ) ) ;
#9741=DIRECTION ( 'NONE',  ( 0.000000000000000000, 0.000000000000000000, 1.000000000000000000 ) ) ;
#9753=DIRECTION ( 'NONE',  ( 0.000000000000000000, -0.000000000000000000, 1.000000000000000000 ) ) ;
#9754=ORIENTED_EDGE ( 'NONE', *, *, #25930, .F. ) ;
#9782=EDGE_CURVE ( 'NONE', #4684, #20354, #30610, .T. ) ;
#9787=AXIS2_PLACEMENT_3D ( 'NONE', #891, #4458, #32771 ) ;
#9792=DIRECTION ( 'NONE',  ( 1.000000000000000000, 0.000000000000000000, 0.000000000000000000 ) ) ;
#9812=EDGE_CURVE ( 'NONE', #35512, #22880, #16362, .T. ) ;
#9817=DIRECTION ( 'NONE',  ( 0.000000000000000000, 0.000000000000000000, 1.000000000000000000 ) ) ;
#9825=CARTESIAN_POINT ( 'NONE',  ( -102.5304832720503185, -102.5304832720485280, 32.55002500000000509 ) ) ;
#9833=ORIENTED_EDGE ( 'NONE', *, *, #5642, .F. ) ;
#9850=DIRECTION ( 'NONE',  ( 0.000000000000000000, -0.000000000000000000, -1.000000000000000000 ) ) ;
#9853=DIRECTION ( 'NONE',  ( -0.000000000000000000, -0.000000000000000000, -1.000000000000000000 ) ) ;
#9886=CARTESIAN_POINT ( 'NONE',  ( -96.90577897536184082, 67.77529820641851188, 32.50000000000000711 ) ) ;
#9899=ORIENTED_EDGE ( 'NONE', *, *, #33865, .F. ) ;
#9905=DIRECTION ( 'NONE',  ( 0.7071067811865489050, 0.7071067811865461294, 0.000000000000000000 ) ) ;
#9908=VERTEX_POINT ( 'NONE', #23644 ) ;
#9911=ORIENTED_EDGE ( 'NONE', *, *, #26763, .F. ) ;
#9924=CARTESIAN_POINT ( 'NONE',  ( 104.8061974404897683, -19.22934205795014151, 32.50000000000000000 ) ) ;
#9926=ADVANCED_FACE ( 'NONE', ( #589 ), #25743, .F. ) ;
#9933=ORIENTED_EDGE ( 'NONE', *, *, #8613, .F. ) ;
#9939=CARTESIAN_POINT ( 'NONE',  ( 145.0000000000000568, -5.056524707326808249E-13, 32.50000000000000000 ) ) ;
#9949=AXIS2_PLACEMENT_3D ( 'NONE', #21939, #33581, #22138 ) ;
#9950=AXIS2_PLACEMENT_3D ( 'NONE', #6389, #14634, #32046 ) ;
#9962=DIRECTION ( 'NONE',  ( 0.000000000000000000, 0.000000000000000000, 1.000000000000000000 ) ) ;
#9966=EDGE_LOOP ( 'NONE', ( #25252, #32098, #34265, #32797 ) ) ;
#10016=DIRECTION ( 'NONE',  ( 1.000000000000000000, 0.000000000000000000, 0.000000000000000000 ) ) ;
#10026=ORIENTED_EDGE ( 'NONE', *, *, #33706, .F. ) ;
#10041=MECHANICAL_DESIGN_GEOMETRIC_PRESENTATION_REPRESENTATION('',(#29690),#21410);
#10045=DIRECTION ( 'NONE',  ( -0.000000000000000000, -0.000000000000000000, 1.000000000000000000 ) ) ;
#10046=DIRECTION ( 'NONE',  ( 1.000000000000000000, 0.000000000000000000, 0.000000000000000000 ) ) ;
#10049=FACE_OUTER_BOUND ( 'NONE', #1920, .T. ) ;
#10074=ORIENTED_EDGE ( 'NONE', *, *, #33427, .T. ) ;
#10078=DIRECTION ( 'NONE',  ( -0.000000000000000000, -0.000000000000000000, -1.000000000000000000 ) ) ;
#10080=ADVANCED_FACE ( 'NONE', ( #13141 ), #26835, .T. ) ;
#10093=AXIS2_PLACEMENT_3D ( 'NONE', #12768, #19345, #36222 ) ;
#10105=ORIENTED_EDGE ( 'NONE', *, *, #5059, .T. ) ;
#10118=EDGE_LOOP ( 'NONE', ( #15682, #4100, #30956, #23538 ) ) ;
#10139=FILL_AREA_STYLE ('',( #30729 ) ) ;
#10149=CARTESIAN_POINT ( 'NONE',  ( -10.49238116876062499, -117.7011972391635908, 32.50000000000000000 ) ) ;
#10159=VECTOR ( 'NONE', #34994, 1000.000000000000000 ) ;
#10204=EDGE_LOOP ( 'NONE', ( #23084, #11515, #5940, #9144 ) ) ;
#10218=CARTESIAN_POINT ( 'NONE',  ( -107.2742589609544410, 47.50000425637879431, 32.50001250000000397 ) ) ;
#10219=CARTESIAN_POINT ( 'NONE',  ( 5.999999999999998224, 145.0000000000000568, 27.50000000000000000 ) ) ;
#10228=ORIENTED_EDGE ( 'NONE', *, *, #31974, .F. ) ;
#10231=CYLINDRICAL_SURFACE ( 'NONE', #9472, 95.00000000000001421 ) ;
#10233=CARTESIAN_POINT ( 'NONE',  ( 37.50000000000000000, 103.4105893997321743, 32.50000000000000000 ) ) ;
#10237=FACE_BOUND ( 'NONE', #3501, .T. ) ;
#10253=EDGE_LOOP ( 'NONE', ( #9027, #24341, #22735, #31264 ) ) ;
#10274=CARTESIAN_POINT ( 'NONE',  ( -94.40806000769299544, 12.15049814296761888, 27.50000000000000000 ) ) ;
#10281=ADVANCED_FACE ( 'NONE', ( #32003 ), #14206, .F. ) ;
#10284=EDGE_LOOP ( 'NONE', ( #28419, #5820, #8804, #13198 ) ) ;
#10291=ORIENTED_EDGE ( 'NONE', *, *, #18340, .F. ) ;
#10301=DIRECTION ( 'NONE',  ( -1.000000000000000000, 3.491481338843133750E-15, 0.000000000000000000 ) ) ;
#10320=CARTESIAN_POINT ( 'NONE',  ( -111.8061974404896262, 19.22934205795090534, 32.50000000000000000 ) ) ;
#10321=DIRECTION ( 'NONE',  ( 1.000000000000000000, 0.000000000000000000, 0.000000000000000000 ) ) ;
#10328=EDGE_CURVE ( 'NONE', #31169, #40, #28995, .T. ) ;
#10344=CIRCLE ( 'NONE', #156, 150.0000000000000284 ) ;
#10358=ORIENTED_EDGE ( 'NONE', *, *, #7003, .T. ) ;
#10378=LINE ( 'NONE', #1214, #29764 ) ;
#10381=CARTESIAN_POINT ( 'NONE',  ( 108.3061974404898820, 19.22934205794938478, 32.50000000000000000 ) ) ;
#10402=ORIENTED_EDGE ( 'NONE', *, *, #18406, .F. ) ;
#10415=CARTESIAN_POINT ( 'NONE',  ( 82.27241335952147949, -47.50000000000039790, 27.50000000000000000 ) ) ;
#10419=CARTESIAN_POINT ( 'NONE',  ( 102.5304832720496080, 102.5304832720492527, 27.50000000000000000 ) ) ;
#10452=VERTEX_POINT ( 'NONE', #901 ) ;
#10453=EDGE_CURVE ( 'NONE', #4684, #35726, #6263, .T. ) ;
#10454=AXIS2_PLACEMENT_3D ( 'NONE', #22811, #25971, #273 ) ;
#10482=CARTESIAN_POINT ( 'NONE',  ( -85.17994309527703933, -72.40128952002849871, 32.50000000000000000 ) ) ;
#10486=ORIENTED_EDGE ( 'NONE', *, *, #25672, .F. ) ;
#10529=CYLINDRICAL_SURFACE ( 'NONE', #986, 3.499999999999996003 ) ;
#10542=AXIS2_PLACEMENT_3D ( 'NONE', #877, #10078, #24317 ) ;
#10544=EDGE_CURVE ( 'NONE', #25010, #25525, #23794, .T. ) ;
#10598=CARTESIAN_POINT ( 'NONE',  ( -102.5304832720481869, 102.5304832720506596, 27.50000000000000000 ) ) ;
#10608=VERTEX_POINT ( 'NONE', #20145 ) ;
#10618=DIRECTION ( 'NONE',  ( 1.000000000000000000, 0.000000000000000000, 0.000000000000000000 ) ) ;
#10624=LINE ( 'NONE', #13245, #11759 ) ;
#10625=CIRCLE ( 'NONE', #34547, 25.00000000000000000 ) ;
#10641=CARTESIAN_POINT ( 'NONE',  ( -81.11590899555835676, 72.50427799314736887, 32.49999999999999289 ) ) ;
#10669=EDGE_LOOP ( 'NONE', ( #7173, #16253, #33902, #33467 ) ) ;
#10681=CARTESIAN_POINT ( 'NONE',  ( 92.89190886694493088, -70.24536753140540668, 32.50000000000000000 ) ) ;
#10688=ORIENTED_EDGE ( 'NONE', *, *, #6728, .F. ) ;
#10708=CARTESIAN_POINT ( 'NONE',  ( -149.8799519615615736, 6.000000000001555200, 27.50000000000000000 ) ) ;
#10715=CARTESIAN_POINT ( 'NONE',  ( 145.0000000000000853, 5.999999999999493738, 32.55002500000000509 ) ) ;
#10727=ORIENTED_EDGE ( 'NONE', *, *, #13, .F. ) ;
#10731=ORIENTED_EDGE ( 'NONE', *, *, #22046, .T. ) ;
#10737=DIRECTION ( 'NONE',  ( 1.000000000000000000, 0.000000000000000000, 0.000000000000000000 ) ) ;
#10741=EDGE_LOOP ( 'NONE', ( #6185, #29782, #5796, #7671 ) ) ;
#10748=VERTEX_POINT ( 'NONE', #815 ) ;
#10752=VECTOR ( 'NONE', #31967, 1000.000000000000000 ) ;
#10756=DIRECTION ( 'NONE',  ( 1.000000000000000000, 0.000000000000000000, 0.000000000000000000 ) ) ;
#10758=CARTESIAN_POINT ( 'NONE',  ( 6.000000000000000000, -149.8799519615616305, 32.55002500000000509 ) ) ;
#10761=ADVANCED_FACE ( 'NONE', ( #14895 ), #643, .T. ) ;
#10779=ORIENTED_EDGE ( 'NONE', *, *, #15148, .T. ) ;
#10800=CARTESIAN_POINT ( 'NONE',  ( 111.8061974404897825, -19.22934205795014151, 32.50000000000000000 ) ) ;
#10807=VERTEX_POINT ( 'NONE', #34598 ) ;
#10812=CARTESIAN_POINT ( 'NONE',  ( -5.999999999999985789, -149.8799519615616305, 27.50000000000000000 ) ) ;
#10817=DIRECTION ( 'NONE',  ( -0.000000000000000000, 0.000000000000000000, -1.000000000000000000 ) ) ;
#10845=LINE ( 'NONE', #5022, #27474 ) ;
#10847=ORIENTED_EDGE ( 'NONE', *, *, #19162, .F. ) ;
#10859=CARTESIAN_POINT ( 'NONE',  ( 106.8646913500057707, -42.81758297416944004, 32.50000000000000000 ) ) ;
#10860=CARTESIAN_POINT ( 'NONE',  ( -78.38327399104142046, -72.20004170604832439, 32.50000000000000711 ) ) ;
#10862=LINE ( 'NONE', #36733, #30993 ) ;
#10869=LINE ( 'NONE', #21579, #9528 ) ;
#10870=ORIENTED_EDGE ( 'NONE', *, *, #35582, .F. ) ;
#10877=CARTESIAN_POINT ( 'NONE',  ( 94.40806000769313755, 12.15049814296589226, 32.50000000000000000 ) ) ;
#10915=AXIS2_PLACEMENT_3D ( 'NONE', #22528, #16904, #5644 ) ;
#10948=VERTEX_POINT ( 'NONE', #15636 ) ;
#10955=ORIENTED_EDGE ( 'NONE', *, *, #21145, .T. ) ;
#10965=DIRECTION ( 'NONE',  ( -1.000000000000000000, 1.082992363797667670E-14, 0.000000000000000000 ) ) ;
#10979=ORIENTED_EDGE ( 'NONE', *, *, #27181, .F. ) ;
#10982=VERTEX_POINT ( 'NONE', #25198 ) ;
#11025=DIRECTION ( 'NONE',  ( 1.000000000000000000, 0.000000000000000000, 0.000000000000000000 ) ) ;
#11030=CARTESIAN_POINT ( 'NONE',  ( 106.2299462780987227, -40.32678999516329554, 32.50000000000000711 ) ) ;
#11065=AXIS2_PLACEMENT_3D ( 'NONE', #5381, #17174, #22612 ) ;
#11084=ORIENTED_EDGE ( 'NONE', *, *, #1998, .T. ) ;
#11090=AXIS2_PLACEMENT_3D ( 'NONE', #17856, #34754, #31727 ) ;
#11096=DIRECTION ( 'NONE',  ( -0.000000000000000000, -0.000000000000000000, 1.000000000000000000 ) ) ;
#11100=CARTESIAN_POINT ( 'NONE',  ( 102.5304832720488832, -102.5304832720499633, 32.55002500000000509 ) ) ;
#11101=DIRECTION ( 'NONE',  ( -0.000000000000000000, -0.000000000000000000, -1.000000000000000000 ) ) ;
#11115=CIRCLE ( 'NONE', #23112, 3.499999999999996003 ) ;
#11122=AXIS2_PLACEMENT_3D ( 'NONE', #3712, #6527, #11410 ) ;
#11138=LINE ( 'NONE', #14137, #23965 ) ;
#11143=EDGE_CURVE ( 'NONE', #17730, #35778, #12179, .T. ) ;
#11208=CIRCLE ( 'NONE', #36973, 3.499999999999996003 ) ;
#11218=EDGE_CURVE ( 'NONE', #18582, #14464, #18464, .T. ) ;
#11224=CARTESIAN_POINT ( 'NONE',  ( -106.4310728746527133, -54.27667806281213103, 32.50000000000000000 ) ) ;
#11226=LINE ( 'NONE', #22471, #3429 ) ;
#11228=FACE_OUTER_BOUND ( 'NONE', #34313, .T. ) ;
#11234=DIRECTION ( 'NONE',  ( -1.000000000000000000, 0.000000000000000000, 0.000000000000000000 ) ) ;
#11247=( NAMED_UNIT ( * ) SI_UNIT ( $, .STERADIAN. ) SOLID_ANGLE_UNIT ( ) );
#11258=EDGE_CURVE ( 'NONE', #11631, #18383, #26286, .T. ) ;
#11294=CARTESIAN_POINT ( 'NONE',  ( 94.55012560584677317, -9.234378588654733377, 27.50000000000000000 ) ) ;
#11307=DIRECTION ( 'NONE',  ( 0.000000000000000000, 0.000000000000000000, 1.000000000000000000 ) ) ;
#11318=CARTESIAN_POINT ( 'NONE',  ( 9.944411252287574499, 118.0778277273563788, 27.49998800000000543 ) ) ;
#11345=DIRECTION ( 'NONE',  ( 1.000000000000000000, 0.000000000000000000, 0.000000000000000000 ) ) ;
#11347=DIRECTION ( 'NONE',  ( -0.000000000000000000, 0.000000000000000000, -1.000000000000000000 ) ) ;
#11348=AXIS2_PLACEMENT_3D ( 'NONE', #20536, #6681, #12660 ) ;
#11349=EDGE_LOOP ( 'NONE', ( #29830, #28988, #33187, #1098 ) ) ;
#11365=CARTESIAN_POINT ( 'NONE',  ( 6.000000000000000000, -145.0000000000000568, 32.55002500000000509 ) ) ;
#11376=CARTESIAN_POINT ( 'NONE',  ( 108.3061974404897825, -19.22934205795014151, 32.50000000000000000 ) ) ;
#11379=AXIS2_PLACEMENT_3D ( 'NONE', #27808, #5507, #14317 ) ;
#11410=DIRECTION ( 'NONE',  ( 1.000000000000000000, 0.000000000000000000, 0.000000000000000000 ) ) ;
#11411=CARTESIAN_POINT ( 'NONE',  ( 5.999999999999947597, -2.132877728683645235E-15, 27.50000000000000000 ) ) ;
#11432=VERTEX_POINT ( 'NONE', #10708 ) ;
#11439=DIRECTION ( 'NONE',  ( 0.000000000000000000, 0.000000000000000000, 1.000000000000000000 ) ) ;
#11455=DIRECTION ( 'NONE',  ( 0.7071067811865389130, -0.7071067811865561215, 0.000000000000000000 ) ) ;
#11461=ORIENTED_EDGE ( 'NONE', *, *, #29393, .T. ) ;
#11467=DIRECTION ( 'NONE',  ( 0.000000000000000000, 0.000000000000000000, 1.000000000000000000 ) ) ;
#11471=ORIENTED_EDGE ( 'NONE', *, *, #28621, .F. ) ;
#11472=ORIENTED_EDGE ( 'NONE', *, *, #5789, .F. ) ;
#11481=DIRECTION ( 'NONE',  ( -0.000000000000000000, -0.000000000000000000, 1.000000000000000000 ) ) ;
#11499=ORIENTED_EDGE ( 'NONE', *, *, #31222, .T. ) ;
#11500=DIRECTION ( 'NONE',  ( 1.000000000000000000, -8.673617379884035472E-16, 0.000000000000000000 ) ) ;
#11515=ORIENTED_EDGE ( 'NONE', *, *, #36729, .F. ) ;
#11517=CARTESIAN_POINT ( 'NONE',  ( -124.4080600076932370, -12.15049814296501829, 32.50000000000000000 ) ) ;
#11530=DIRECTION ( 'NONE',  ( 1.000000000000000000, 0.000000000000000000, 0.000000000000000000 ) ) ;
#11548=DIRECTION ( 'NONE',  ( -0.7071067811865487940, -0.7071067811865463515, 0.000000000000000000 ) ) ;
#11567=FACE_OUTER_BOUND ( 'NONE', #13450, .T. ) ;
#11569=CARTESIAN_POINT ( 'NONE',  ( -107.2751058113818203, -48.40472568396508279, 32.49999999999998579 ) ) ;
#11584=EDGE_LOOP ( 'NONE', ( #3640, #30506 ) ) ;
#11585=VERTEX_POINT ( 'NONE', #9154 ) ;
#11605=CARTESIAN_POINT ( 'NONE',  ( -37.50000000000000000, 103.4105893997321743, 27.50000000000000000 ) ) ;
#11613=LINE ( 'NONE', #23068, #12999 ) ;
#11631=VERTEX_POINT ( 'NONE', #3007 ) ;
#11632=CARTESIAN_POINT ( 'NONE',  ( 145.0000000000000284, -6.000000000000504485, 32.55002500000000509 ) ) ;
#11640=AXIS2_PLACEMENT_3D ( 'NONE', #1293, #15360, #15918 ) ;
#11650=CYLINDRICAL_SURFACE ( 'NONE', #36078, 25.00000000000000000 ) ;
#11653=CIRCLE ( 'NONE', #35039, 95.00000000000001421 ) ;
#11654=EDGE_CURVE ( 'NONE', #4310, #6715, #3423, .T. ) ;
#11679=CARTESIAN_POINT ( 'NONE',  ( 8.711340810219693864, -118.4423164015428256, 32.50000000000000711 ) ) ;
#11697=ORIENTED_EDGE ( 'NONE', *, *, #5340, .F. ) ;
#11705=CIRCLE ( 'NONE', #30291, 150.0000000000000284 ) ;
#11723=VECTOR ( 'NONE', #16209, 1000.000000000000000 ) ;
#11729=ORIENTED_EDGE ( 'NONE', *, *, #32497, .T. ) ;
#11735=FACE_OUTER_BOUND ( 'NONE', #17421, .T. ) ;
#11750=ORIENTED_EDGE ( 'NONE', *, *, #27556, .F. ) ;
#11754=CARTESIAN_POINT ( 'NONE',  ( -102.5304832720503185, -102.5304832720485280, 27.50000000000000000 ) ) ;
#11759=VECTOR ( 'NONE', #24692, 1000.000000000000000 ) ;
#11761=DIRECTION ( 'NONE',  ( 0.7071067811865414665, -0.7071067811865536790, -0.000000000000000000 ) ) ;
#11775=CLOSED_SHELL ( 'NONE', ( #33604, #34142, #3962, #15826, #19284, #33301, #7947, #2031, #36687, #2661, #10281, #32917, #7309, #35097, #15070, #4725, #30656, #23171, #19066, #14023, #16154, #18454, #36672, #29823, #33996, #6065, #10080, #36104, #15073, #13078, #26030, #2566, #19872, #14429, #14633, #6542, #5103, #6176, #17817, #654, #5106, #36704, #8282, #12953, #12007, #4272, #35436, #10761, #14375, #19961, #30173, #29363, #2219, #12487, #26316, #7116, #27552, #4331, #21100, #15115, #21843, #28450, #31480, #34181, #29356, #13920, #7530, #28891, #1972, #18720, #2271, #36617, #24782, #28348, #31788, #2783, #9926, #26505, #23687, #1636, #16196, #37090, #21934, #32552, #6992, #25018, #29594, #36608, #9622, #12297 ) ) ;
#11777=DIRECTION ( 'NONE',  ( 1.000000000000000000, 0.000000000000000000, 0.000000000000000000 ) ) ;
#11779=( LENGTH_UNIT ( ) NAMED_UNIT ( * ) SI_UNIT ( .MILLI., .METRE. ) );
#11780=AXIS2_PLACEMENT_3D ( 'NONE', #26138, #34950, #9071 ) ;
#11796=FACE_OUTER_BOUND ( 'NONE', #10284, .T. ) ;
#11817=CARTESIAN_POINT ( 'NONE',  ( 74.30619744048946984, -84.18124734178287838, 32.50000000000000000 ) ) ;
#11818=ORIENTED_EDGE ( 'NONE', *, *, #32675, .F. ) ;
#11832=VECTOR ( 'NONE', #785, 1000.000000000000000 ) ;
#11835=ORIENTED_EDGE ( 'NONE', *, *, #2880, .F. ) ;
#11873=CARTESIAN_POINT ( 'NONE',  ( -9.904827271909082853, -117.9629806292090279, 32.50000000000000711 ) ) ;
#11883=DIRECTION ( 'NONE',  ( 0.000000000000000000, 0.000000000000000000, 1.000000000000000000 ) ) ;
#11887=CARTESIAN_POINT ( 'NONE',  ( -102.5304832720481869, 102.5304832720506596, 32.55002500000000509 ) ) ;
#11900=CIRCLE ( 'NONE', #7130, 3.500000000000003109 ) ;
#11906=CARTESIAN_POINT ( 'NONE',  ( -101.4249800177810812, 31.43204461044035725, 27.50000000000000000 ) ) ;
#11911=EDGE_CURVE ( 'NONE', #3013, #10982, #540, .T. ) ;
#11932=EDGE_CURVE ( 'NONE', #9158, #18582, #10845, .T. ) ;
#11934=AXIS2_PLACEMENT_3D ( 'NONE', #5375, #27667, #2374 ) ;
#11937=EDGE_LOOP ( 'NONE', ( #15481, #31902, #19447, #28043 ) ) ;
#11955=CARTESIAN_POINT ( 'NONE',  ( 0.000000000000000000, 0.000000000000000000, 27.50000000000000000 ) ) ;
#11956=CIRCLE ( 'NONE', #26932, 30.00000000000000000 ) ;
#11964=VERTEX_POINT ( 'NONE', #19654 ) ;
#11971=DIRECTION ( 'NONE',  ( 0.000000000000000000, 0.000000000000000000, 1.000000000000000000 ) ) ;
#11974=ORIENTED_EDGE ( 'NONE', *, *, #9782, .T. ) ;
#11976=AXIS2_PLACEMENT_3D ( 'NONE', #21915, #4686, #33362 ) ;
#11980=DIRECTION ( 'NONE',  ( 1.000000000000000000, 0.000000000000000000, 0.000000000000000000 ) ) ;
#11984=CARTESIAN_POINT ( 'NONE',  ( 107.1784174493373172, 49.76392998123883160, 32.50000000000000000 ) ) ;
#11985=FACE_OUTER_BOUND ( 'NONE', #22575, .T. ) ;
#11994=ORIENTED_EDGE ( 'NONE', *, *, #23714, .F. ) ;
#12007=ADVANCED_FACE ( 'NONE', ( #23007 ), #5578, .T. ) ;
#12011=CARTESIAN_POINT ( 'NONE',  ( -4.242640687119282106, 4.242640687119296317, 27.50000000000000000 ) ) ;
#12026=PLANE ( 'NONE',  #36274 ) ;
#12027=EDGE_CURVE ( 'NONE', #16830, #10807, #14203, .T. ) ;
#12038=ORIENTED_EDGE ( 'NONE', *, *, #6612, .F. ) ;
#12055=CARTESIAN_POINT ( 'NONE',  ( -108.3061974404896262, 19.22934205795090534, 27.50000000000000000 ) ) ;
#12064=CARTESIAN_POINT ( 'NONE',  ( 98.28784258492957804, -106.7731239591692116, 32.55002500000000509 ) ) ;
#12077=ORIENTED_EDGE ( 'NONE', *, *, #26802, .F. ) ;
#12078=DIRECTION ( 'NONE',  ( 0.7071067811865389130, -0.7071067811865561215, 0.000000000000000000 ) ) ;
#12090=DIRECTION ( 'NONE',  ( -0.000000000000000000, -0.000000000000000000, 1.000000000000000000 ) ) ;
#12096=EDGE_CURVE ( 'NONE', #19856, #31753, #20546, .T. ) ;
#12140=AXIS2_PLACEMENT_3D ( 'NONE', #17330, #5520, #19944 ) ;
#12143=CIRCLE ( 'NONE', #33129, 150.0000000000000284 ) ;
#12147=VERTEX_POINT ( 'NONE', #4068 ) ;
#12149=CARTESIAN_POINT ( 'NONE',  ( 0.000000000000000000, 95.00000000000001421, 32.50000000000000000 ) ) ;
#12179=LINE ( 'NONE', #23469, #6469 ) ;
#12189=CARTESIAN_POINT ( 'NONE',  ( 0.000000000000000000, 0.000000000000000000, 32.50000000000000000 ) ) ;
#12257=DIRECTION ( 'NONE',  ( 1.000000000000000000, 0.000000000000000000, 0.000000000000000000 ) ) ;
#12264=LINE ( 'NONE', #3846, #3337 ) ;
#12272=EDGE_CURVE ( 'NONE', #36161, #27930, #35309, .T. ) ;
#12290=CIRCLE ( 'NONE', #20682, 95.00000000000001421 ) ;
#12293=EDGE_CURVE ( 'NONE', #22692, #460, #18547, .T. ) ;
#12297=ADVANCED_FACE ( 'NONE', ( #16252 ), #16421, .F. ) ;
#12307=ORIENTED_EDGE ( 'NONE', *, *, #23377, .F. ) ;
#12311=EDGE_CURVE ( 'NONE', #11585, #6228, #31688, .T. ) ;
#12346=CARTESIAN_POINT ( 'NONE',  ( 98.21838448168142577, 66.76540064347040015, 32.50000000000000711 ) ) ;
#12347=DIRECTION ( 'NONE',  ( 1.082992363797667670E-14, 1.000000000000000000, 0.000000000000000000 ) ) ;
#12356=ORIENTED_EDGE ( 'NONE', *, *, #24105, .F. ) ;
#12358=CARTESIAN_POINT ( 'NONE',  ( 95.00000000000001421, 0.000000000000000000, 27.50000000000000000 ) ) ;
#12363=DIRECTION ( 'NONE',  ( 0.000000000000000000, 0.000000000000000000, 1.000000000000000000 ) ) ;
#12406=ORIENTED_EDGE ( 'NONE', *, *, #33798, .F. ) ;
#12429=AXIS2_PLACEMENT_3D ( 'NONE', #34124, #5795, #19854 ) ;
#12433=ORIENTED_EDGE ( 'NONE', *, *, #5338, .T. ) ;
#12435=CIRCLE ( 'NONE', #27416, 5.999999999999999112 ) ;
#12436=DIRECTION ( 'NONE',  ( 1.000000000000000000, 0.000000000000000000, 0.000000000000000000 ) ) ;
#12456=FACE_OUTER_BOUND ( 'NONE', #23705, .T. ) ;
#12458=CARTESIAN_POINT ( 'NONE',  ( 6.497954182785949224E-14, 5.999999999999947597, 27.50000000000000000 ) ) ;
#12462=ORIENTED_EDGE ( 'NONE', *, *, #23758, .F. ) ;
#12469=CARTESIAN_POINT ( 'NONE',  ( -107.2742747693529566, -47.50000423952285900, 32.50001250000000397 ) ) ;
#12478=CARTESIAN_POINT ( 'NONE',  ( 37.50000000000000000, -103.4105893997321743, 32.50000000000000000 ) ) ;
#12487=ADVANCED_FACE ( 'NONE', ( #20504 ), #19972, .T. ) ;
#12509=AXIS2_PLACEMENT_3D ( 'NONE', #35601, #23587, #9713 ) ;
#12514=AXIS2_PLACEMENT_3D ( 'NONE', #31429, #118, #11548 ) ;
#12530=DIRECTION ( 'NONE',  ( 0.7071067811865461294, -0.7071067811865489050, 0.000000000000000000 ) ) ;
#12544=FACE_OUTER_BOUND ( 'NONE', #21221, .T. ) ;
#12547=CARTESIAN_POINT ( 'NONE',  ( 102.9785771442050333, 33.47437999733440250, 32.50000000000000000 ) ) ;
#12548=CIRCLE ( 'NONE', #7780, 30.00000000000000000 ) ;
#12565=DIRECTION ( 'NONE',  ( 1.000000000000000000, 0.000000000000000000, 0.000000000000000000 ) ) ;
#12566=ORIENTED_EDGE ( 'NONE', *, *, #36316, .F. ) ;
#12568=CARTESIAN_POINT ( 'NONE',  ( -51.68138994340220904, -113.8157894736842053, 27.50000000000000000 ) ) ;
#12569=DIRECTION ( 'NONE',  ( 1.000000000000000000, 0.000000000000000000, 0.000000000000000000 ) ) ;
#12573=DIRECTION ( 'NONE',  ( 0.000000000000000000, 0.000000000000000000, 1.000000000000000000 ) ) ;
#12587=DIRECTION ( 'NONE',  ( 1.000000000000000000, 0.000000000000000000, 0.000000000000000000 ) ) ;
#12590=EDGE_LOOP ( 'NONE', ( #6047, #3207, #6107, #15619 ) ) ;
#12606=ORIENTED_EDGE ( 'NONE', *, *, #806, .T. ) ;
#12608=ORIENTED_EDGE ( 'NONE', *, *, #11258, .F. ) ;
#12624=CARTESIAN_POINT ( 'NONE',  ( -82.27241335952211898, -47.49999999999924682, 32.50002500000000083 ) ) ;
#12647=VERTEX_POINT ( 'NONE', #3655 ) ;
#12648=ORIENTED_EDGE ( 'NONE', *, *, #12293, .T. ) ;
#12660=DIRECTION ( 'NONE',  ( 1.000000000000000000, 0.000000000000000000, 0.000000000000000000 ) ) ;
#12685=CARTESIAN_POINT ( 'NONE',  ( -77.93337651276257816, 72.12094976675054170, 32.50001250000000397 ) ) ;
#12688=ORIENTED_EDGE ( 'NONE', *, *, #3206, .T. ) ;
#12710=ORIENTED_EDGE ( 'NONE', *, *, #9671, .T. ) ;
#12717=VERTEX_POINT ( 'NONE', #9324 ) ;
#12721=EDGE_CURVE ( 'NONE', #4461, #27222, #32340, .T. ) ;
#12729=DIRECTION ( 'NONE',  ( 1.000000000000000000, 0.000000000000000000, 0.000000000000000000 ) ) ;
#12737=DIRECTION ( 'NONE',  ( -0.000000000000000000, -0.000000000000000000, -1.000000000000000000 ) ) ;
#12738=LINE ( 'NONE', #6587, #16547 ) ;
#12740=VERTEX_POINT ( 'NONE', #29756 ) ;
#12744=ORIENTED_EDGE ( 'NONE', *, *, #32087, .F. ) ;
#12754=DIRECTION ( 'NONE',  ( -0.7071067811865388020, 0.7071067811865563435, 0.000000000000000000 ) ) ;
#12768=CARTESIAN_POINT ( 'NONE',  ( 108.3061974404898820, 19.22934205794938478, 32.50000000000000000 ) ) ;
#12776=LINE ( 'NONE', #23882, #17800 ) ;
#12803=DIRECTION ( 'NONE',  ( 0.000000000000000000, 0.000000000000000000, 1.000000000000000000 ) ) ;
#12830=EDGE_CURVE ( 'NONE', #27264, #20315, #24813, .T. ) ;
#12835=CARTESIAN_POINT ( 'NONE',  ( -106.7731239591675205, 98.28784258493143966, 32.50000000000000000 ) ) ;
#12849=DIRECTION ( 'NONE',  ( 1.000000000000000000, 0.000000000000000000, 0.000000000000000000 ) ) ;
#12855=CARTESIAN_POINT ( 'NONE',  ( 96.53048327204960799, 102.5304832720492527, 32.55002500000000509 ) ) ;
#12859=ORIENTED_EDGE ( 'NONE', *, *, #23789, .F. ) ;
#12866=ORIENTED_EDGE ( 'NONE', *, *, #5059, .F. ) ;
#12868=PLANE ( 'NONE',  #1677 ) ;
#12870=CARTESIAN_POINT ( 'NONE',  ( -99.75152572807942875, 65.47112307816239252, 32.50000000000000000 ) ) ;
#12876=EDGE_CURVE ( 'NONE', #23345, #31169, #20668, .T. ) ;
#12904=ORIENTED_EDGE ( 'NONE', *, *, #29292, .T. ) ;
#12921=DIRECTION ( 'NONE',  ( 1.000000000000000000, 0.000000000000000000, 0.000000000000000000 ) ) ;
#12934=CIRCLE ( 'NONE', #14144, 3.499999999999996003 ) ;
#12953=ADVANCED_FACE ( 'NONE', ( #25945 ), #8883, .T. ) ;
#12962=AXIS2_PLACEMENT_3D ( 'NONE', #28956, #22289, #11025 ) ;
#12966=PRODUCT_DEFINITION_FORMATION_WITH_SPECIFIED_SOURCE ( 'ANY', '', #20242, .NOT_KNOWN. ) ;
#12971=EDGE_LOOP ( 'NONE', ( #35830, #29548, #27182, #5174 ) ) ;
#12986=AXIS2_PLACEMENT_3D ( 'NONE', #7641, #27513, #35773 ) ;
#12988=ORIENTED_EDGE ( 'NONE', *, *, #27860, .T. ) ;
#12991=CIRCLE ( 'NONE', #16596, 3.500000000000003109 ) ;
#12999=VECTOR ( 'NONE', #34516, 1000.000000000000000 ) ;
#13010=CIRCLE ( 'NONE', #29783, 30.00000000000000000 ) ;
#13025=VERTEX_POINT ( 'NONE', #31370 ) ;
#13034=CARTESIAN_POINT ( 'NONE',  ( 5.999999999999947597, -2.132877728683645235E-15, 32.50000000000000000 ) ) ;
#13041=DIRECTION ( 'NONE',  ( 1.000000000000000000, 0.000000000000000000, 0.000000000000000000 ) ) ;
#13042=DIRECTION ( 'NONE',  ( -0.7071067811865439090, 0.7071067811865512365, 0.000000000000000000 ) ) ;
#13060=VERTEX_POINT ( 'NONE', #21228 ) ;
#13066=CARTESIAN_POINT ( 'NONE',  ( -108.3061974404900241, -19.22934205794863516, 32.50000000000000000 ) ) ;
#13069=CARTESIAN_POINT ( 'NONE',  ( 149.8799519615616589, 5.999999999999476863, 32.50000000000000000 ) ) ;
#13078=ADVANCED_FACE ( 'NONE', ( #24433 ), #35502, .F. ) ;
#13081=EDGE_LOOP ( 'NONE', ( #35062, #31290 ) ) ;
#13086=AXIS2_PLACEMENT_3D ( 'NONE', #20079, #5480, #19901 ) ;
#13092=EDGE_CURVE ( 'NONE', #13968, #27821, #12776, .T. ) ;
#13104=CARTESIAN_POINT ( 'NONE',  ( -107.2777746127022453, 46.05181527023793819, 32.50000000000000711 ) ) ;
#13122=AXIS2_PLACEMENT_3D ( 'NONE', #25653, #25276, #5760 ) ;
#13128=ORIENTED_EDGE ( 'NONE', *, *, #26345, .F. ) ;
#13130=CARTESIAN_POINT ( 'NONE',  ( 0.000000000000000000, 0.000000000000000000, 27.50000000000000000 ) ) ;
#13141=FACE_OUTER_BOUND ( 'NONE', #13263, .T. ) ;
#13162=CARTESIAN_POINT ( 'NONE',  ( -77.93343913441597692, 72.12058696850911588, 27.50000000000000000 ) ) ;
#13175=CARTESIAN_POINT ( 'NONE',  ( -104.3563124639471908, -35.61515136444246821, 32.49999999999999289 ) ) ;
#13181=EDGE_CURVE ( 'NONE', #20872, #31806, #30387, .T. ) ;
#13183=ORIENTED_EDGE ( 'NONE', *, *, #16539, .F. ) ;
#13185=LINE ( 'NONE', #30430, #20190 ) ;
#13192=AXIS2_PLACEMENT_3D ( 'NONE', #37019, #25938, #23316 ) ;
#13198=ORIENTED_EDGE ( 'NONE', *, *, #23377, .T. ) ;
#13227=FACE_BOUND ( 'NONE', #25637, .T. ) ;
#13231=EDGE_CURVE ( 'NONE', #3923, #24921, #36863, .T. ) ;
#13244=CARTESIAN_POINT ( 'NONE',  ( 110.2237710830529664, -101.7384897088154929, 32.55002500000000509 ) ) ;
#13245=CARTESIAN_POINT ( 'NONE',  ( 77.93343913441647430, -72.12058696850856165, 32.50002500000000083 ) ) ;
#13247=ORIENTED_EDGE ( 'NONE', *, *, #35219, .F. ) ;
#13259=VERTEX_POINT ( 'NONE', #33426 ) ;
#13263=EDGE_LOOP ( 'NONE', ( #10979, #14888, #24846, #2826 ) ) ;
#13265=VERTEX_POINT ( 'NONE', #7359 ) ;
#13275=DIRECTION ( 'NONE',  ( 0.000000000000000000, 0.000000000000000000, 1.000000000000000000 ) ) ;
#13276=VERTEX_POINT ( 'NONE', #16355 ) ;
#13280=ORIENTED_EDGE ( 'NONE', *, *, #32087, .T. ) ;
#13287=ORIENTED_EDGE ( 'NONE', *, *, #34712, .T. ) ;
#13290=EDGE_CURVE ( 'NONE', #10452, #28544, #1124, .T. ) ;
#13306=EDGE_CURVE ( 'NONE', #3560, #4570, #35937, .T. ) ;
#13309=EDGE_CURVE ( 'NONE', #16830, #9234, #34525, .T. ) ;
#13311=VERTEX_POINT ( 'NONE', #17086 ) ;
#13324=PLANE ( 'NONE',  #13586 ) ;
#13329=ORIENTED_EDGE ( 'NONE', *, *, #806, .F. ) ;
#13333=ORIENTED_EDGE ( 'NONE', *, *, #6612, .T. ) ;
#13345=VERTEX_POINT ( 'NONE', #11817 ) ;
#13349=VERTEX_POINT ( 'NONE', #14079 ) ;
#13351=DIRECTION ( 'NONE',  ( 0.000000000000000000, 0.000000000000000000, 1.000000000000000000 ) ) ;
#13361=DIRECTION ( 'NONE',  ( -0.000000000000000000, -0.000000000000000000, -1.000000000000000000 ) ) ;
#13392=EDGE_CURVE ( 'NONE', #13968, #1946, #35851, .T. ) ;
#13430=ORIENTED_EDGE ( 'NONE', *, *, #1950, .T. ) ;
#13444=EDGE_CURVE ( 'NONE', #8665, #13345, #17299, .T. ) ;
#13450=EDGE_LOOP ( 'NONE', ( #19098, #2990, #8186, #16908 ) ) ;
#13456=EDGE_CURVE ( 'NONE', #16882, #1598, #19108, .T. ) ;
#13498=EDGE_CURVE ( 'NONE', #3789, #24921, #32440, .T. ) ;
#13527=DIRECTION ( 'NONE',  ( 0.000000000000000000, 0.000000000000000000, 1.000000000000000000 ) ) ;
#13556=AXIS2_PLACEMENT_3D ( 'NONE', #17439, #563, #6019 ) ;
#13586=AXIS2_PLACEMENT_3D ( 'NONE', #10715, #16339, #36761 ) ;
#13588=VECTOR ( 'NONE', #34706, 1000.000000000000000 ) ;
#13591=AXIS2_PLACEMENT_3D ( 'NONE', #42, #19741, #36791 ) ;
#13592=DIRECTION ( 'NONE',  ( 1.000000000000000000, 0.000000000000000000, 0.000000000000000000 ) ) ;
#13611=CARTESIAN_POINT ( 'NONE',  ( -37.50000000000000000, 103.4105893997321743, 27.50000000000000000 ) ) ;
#13612=VECTOR ( 'NONE', #7216, 1000.000000000000000 ) ;
#13629=DIRECTION ( 'NONE',  ( -0.000000000000000000, 0.000000000000000000, -1.000000000000000000 ) ) ;
#13643=EDGE_CURVE ( 'NONE', #27222, #28579, #10869, .T. ) ;
#13675=CARTESIAN_POINT ( 'NONE',  ( 96.68603628058367860, -67.93726725791121623, 32.50000000000000711 ) ) ;
#13691=ORIENTED_EDGE ( 'NONE', *, *, #22232, .T. ) ;
#13694=AXIS2_PLACEMENT_3D ( 'NONE', #12055, #26144, #31577 ) ;
#13718=CARTESIAN_POINT ( 'NONE',  ( -2.308176576174226117E-14, -5.999999999999947597, 32.50000000000000000 ) ) ;
#13732=VERTEX_POINT ( 'NONE', #25858 ) ;
#13741=ORIENTED_EDGE ( 'NONE', *, *, #35933, .T. ) ;
#13747=ORIENTED_EDGE ( 'NONE', *, *, #28124, .T. ) ;
#13755=DIRECTION ( 'NONE',  ( 1.000000000000000000, 0.000000000000000000, 0.000000000000000000 ) ) ;
#13763=CIRCLE ( 'NONE', #25739, 150.0000000000000284 ) ;
#13764=EDGE_CURVE ( 'NONE', #25525, #12740, #26282, .T. ) ;
#13780=FACE_OUTER_BOUND ( 'NONE', #7926, .T. ) ;
#13786=CARTESIAN_POINT ( 'NONE',  ( 101.4249800177814933, 31.43204461043894327, 32.50002500000000083 ) ) ;
#13787=ORIENTED_EDGE ( 'NONE', *, *, #21790, .F. ) ;
#13801=DIRECTION ( 'NONE',  ( -0.000000000000000000, -0.000000000000000000, -1.000000000000000000 ) ) ;
#13842=DIRECTION ( 'NONE',  ( 1.000000000000000000, 0.000000000000000000, 0.000000000000000000 ) ) ;
#13870=SURFACE_SIDE_STYLE ('',( #9411 ) ) ;
#13873=AXIS2_PLACEMENT_3D ( 'NONE', #37047, #23348, #34786 ) ;
#13881=DIRECTION ( 'NONE',  ( -1.000000000000000000, 3.491481338843133750E-15, 0.000000000000000000 ) ) ;
#13886=CARTESIAN_POINT ( 'NONE',  ( -111.8061974404900241, -19.22934205794863516, 32.50000000000000000 ) ) ;
#13892=ORIENTED_EDGE ( 'NONE', *, *, #13764, .F. ) ;
#13896=ORIENTED_EDGE ( 'NONE', *, *, #1607, .T. ) ;
#13920=ADVANCED_FACE ( 'NONE', ( #3545 ), #17774, .F. ) ;
#13932=CARTESIAN_POINT ( 'NONE',  ( -21.38228473677787278, 108.2013388413266739, 27.49998800000000188 ) ) ;
#13937=DIRECTION ( 'NONE',  ( 1.000000000000000000, 0.000000000000000000, 0.000000000000000000 ) ) ;
#13950=CARTESIAN_POINT ( 'NONE',  ( 17.74159560741759378, -112.6248466129485735, 32.50000000000000000 ) ) ;
#13951=EDGE_LOOP ( 'NONE', ( #9899, #12038, #32192, #11471 ) ) ;
#13957=ORIENTED_EDGE ( 'NONE', *, *, #13231, .T. ) ;
#13963=CARTESIAN_POINT ( 'NONE',  ( -101.4249800177810812, 31.43204461044035725, 32.50002500000000083 ) ) ;
#13968=VERTEX_POINT ( 'NONE', #7278 ) ;
#13974=VECTOR ( 'NONE', #34238, 1000.000000000000000 ) ;
#13978=CARTESIAN_POINT ( 'NONE',  ( 70.80619744049005249, 84.18124734178236679, 32.50000000000000000 ) ) ;
#14009=CARTESIAN_POINT ( 'NONE',  ( 104.8061974404897683, -19.22934205795014151, 32.50000000000000000 ) ) ;
#14023=ADVANCED_FACE ( 'NONE', ( #21530 ), #19641, .F. ) ;
#14025=CARTESIAN_POINT ( 'NONE',  ( 105.8340997644729953, -39.11257430625002485, 32.50000000000000000 ) ) ;
#14026=CARTESIAN_POINT ( 'NONE',  ( -103.1654966073423481, -61.26087114250804433, 32.50000000000000000 ) ) ;
#14028=CYLINDRICAL_SURFACE ( 'NONE', #20842, 150.0000000000000284 ) ;
#14052=ORIENTED_EDGE ( 'NONE', *, *, #11932, .F. ) ;
#14059=AXIS2_PLACEMENT_3D ( 'NONE', #28784, #5733, #34616 ) ;
#14076=CARTESIAN_POINT ( 'NONE',  ( 106.7731239591682026, -98.28784258493070070, 32.55002500000000509 ) ) ;
#14079=CARTESIAN_POINT ( 'NONE',  ( -55.27226924886181791, -77.26562141134519379, 32.50000000000000000 ) ) ;
#14094=DIRECTION ( 'NONE',  ( 1.000000000000000000, 0.000000000000000000, 0.000000000000000000 ) ) ;
#14111=DIRECTION ( 'NONE',  ( 0.000000000000000000, 0.000000000000000000, 1.000000000000000000 ) ) ;
#14120=CYLINDRICAL_SURFACE ( 'NONE', #30295, 3.499999999999996003 ) ;
#14137=CARTESIAN_POINT ( 'NONE',  ( -4.242640687119282106, 4.242640687119296317, 32.50000000000000000 ) ) ;
#14140=ORIENTED_EDGE ( 'NONE', *, *, #33593, .T. ) ;
#14144=AXIS2_PLACEMENT_3D ( 'NONE', #17655, #6609, #26655 ) ;
#14168=FACE_OUTER_BOUND ( 'NONE', #1188, .T. ) ;
#14185=CARTESIAN_POINT ( 'NONE',  ( -101.7384897088135887, 110.2237710830547286, 27.50000000000000000 ) ) ;
#14203=LINE ( 'NONE', #17211, #35891 ) ;
#14206=CYLINDRICAL_SURFACE ( 'NONE', #36226, 3.499999999999996003 ) ;
#14212=ORIENTED_EDGE ( 'NONE', *, *, #24723, .T. ) ;
#14217=EDGE_CURVE ( 'NONE', #30663, #13265, #29716, .T. ) ;
#14220=CARTESIAN_POINT ( 'NONE',  ( 78.56323661778957046, -72.23156435200252190, 32.50000000000000000 ) ) ;
#14223=LINE ( 'NONE', #29002, #36387 ) ;
#14224=VECTOR ( 'NONE', #13629, 1000.000000000000000 ) ;
#14225=AXIS2_PLACEMENT_3D ( 'NONE', #24258, #26901, #27247 ) ;
#14249=CARTESIAN_POINT ( 'NONE',  ( 77.93337901593585570, 72.12093275448846441, 32.50001250000000397 ) ) ;
#14263=CIRCLE ( 'NONE', #10093, 3.500000000000003109 ) ;
#14273=CARTESIAN_POINT ( 'NONE',  ( 74.30619744048946984, -84.18124734178287838, 27.50000000000000000 ) ) ;
#14290=CARTESIAN_POINT ( 'NONE',  ( -6.000000000000000000, 0.000000000000000000, 32.50000000000000000 ) ) ;
#14313=CYLINDRICAL_SURFACE ( 'NONE', #20225, 3.499999999999996003 ) ;
#14317=DIRECTION ( 'NONE',  ( 1.000000000000000000, 0.000000000000000000, 0.000000000000000000 ) ) ;
#14319=DIRECTION ( 'NONE',  ( -0.000000000000000000, -0.000000000000000000, 1.000000000000000000 ) ) ;
#14340=AXIS2_PLACEMENT_3D ( 'NONE', #35253, #11971, #32010 ) ;
#14347=EDGE_CURVE ( 'NONE', #10807, #30623, #6678, .T. ) ;
#14375=ADVANCED_FACE ( 'NONE', ( #32529 ), #6846, .T. ) ;
#14376=LINE ( 'NONE', #28797, #8674 ) ;
#14408=CARTESIAN_POINT ( 'NONE',  ( 0.000000000000000000, 0.000000000000000000, 27.50000000000000000 ) ) ;
#14410=CARTESIAN_POINT ( 'NONE',  ( 0.000000000000000000, 0.000000000000000000, 27.50000000000000000 ) ) ;
#14417=DIRECTION ( 'NONE',  ( 0.000000000000000000, 0.000000000000000000, 1.000000000000000000 ) ) ;
#14429=ADVANCED_FACE ( 'NONE', ( #35557, #7794, #27095, #22041, #13227, #10237, #7414, #21665, #32723, #30649, #36106, #21840, #10049, #21284 ), #33093, .F. ) ;
#14433=ORIENTED_EDGE ( 'NONE', *, *, #261, .T. ) ;
#14456=EDGE_CURVE ( 'NONE', #30623, #9129, #34140, .T. ) ;
#14461=DIRECTION ( 'NONE',  ( -0.000000000000000000, -0.000000000000000000, 1.000000000000000000 ) ) ;
#14464=VERTEX_POINT ( 'NONE', #28574 ) ;
#14466=LINE ( 'NONE', #14290, #29051 ) ;
#14468=DIRECTION ( 'NONE',  ( 1.000000000000000000, 0.000000000000000000, 0.000000000000000000 ) ) ;
#14469=ORIENTED_EDGE ( 'NONE', *, *, #19168, .F. ) ;
#14501=EDGE_LOOP ( 'NONE', ( #10228, #21332, #11974, #24966 ) ) ;
#14504=EDGE_CURVE ( 'NONE', #35512, #23824, #25786, .T. ) ;
#14508=ORIENTED_EDGE ( 'NONE', *, *, #2880, .T. ) ;
#14512=CARTESIAN_POINT ( 'NONE',  ( -22.49962511848374902, -105.9192538511173041, 32.50000000000000711 ) ) ;
#14541=VERTEX_POINT ( 'NONE', #36484 ) ;
#14547=PRODUCT_DEFINITION_SHAPE ( 'NONE', 'NONE',  #6997 ) ;
#14548=CARTESIAN_POINT ( 'NONE',  ( -77.93343913441597692, 72.12058696850911588, 32.50002500000000083 ) ) ;
#14550=DIRECTION ( 'NONE',  ( 0.000000000000000000, 0.000000000000000000, 1.000000000000000000 ) ) ;
#14558=EDGE_CURVE ( 'NONE', #6052, #2614, #11138, .T. ) ;
#14566=EDGE_CURVE ( 'NONE', #6228, #10748, #26661, .T. ) ;
#14588=ORIENTED_EDGE ( 'NONE', *, *, #11218, .T. ) ;
#14602=ORIENTED_EDGE ( 'NONE', *, *, #13764, .T. ) ;
#14610=CIRCLE ( 'NONE', #26603, 24.99999999999999289 ) ;
#14616=CARTESIAN_POINT ( 'NONE',  ( -74.30619744048887299, 84.18124734178336155, 32.50000000000000000 ) ) ;
#14628=CARTESIAN_POINT ( 'NONE',  ( 74.30619744048946984, -84.18124734178287838, 32.50000000000000000 ) ) ;
#14633=ADVANCED_FACE ( 'NONE', ( #34944 ), #32107, .T. ) ;
#14634=DIRECTION ( 'NONE',  ( 0.000000000000000000, 0.000000000000000000, 1.000000000000000000 ) ) ;
#14636=CARTESIAN_POINT ( 'NONE',  ( -74.30619744048887299, 84.18124734178336155, 27.50000000000000000 ) ) ;
#14639=EDGE_CURVE ( 'NONE', #12147, #6042, #35141, .T. ) ;
#14663=CARTESIAN_POINT ( 'NONE',  ( 74.30619744049005249, 84.18124734178236679, 32.50000000000000000 ) ) ;
#14677=DIRECTION ( 'NONE',  ( 1.000000000000000000, 0.000000000000000000, 0.000000000000000000 ) ) ;
#14684=CARTESIAN_POINT ( 'NONE',  ( -5.703708899247954101, -119.5207621440044790, 32.50000000000001421 ) ) ;
#14698=CARTESIAN_POINT ( 'NONE',  ( 34.00000000000000000, 103.4105893997321743, 32.50000000000000000 ) ) ;
#14710=DIRECTION ( 'NONE',  ( 1.000000000000000000, 0.000000000000000000, 0.000000000000000000 ) ) ;
#14716=VECTOR ( 'NONE', #29916, 1000.000000000000000 ) ;
#14721=DIRECTION ( 'NONE',  ( 0.000000000000000000, 0.000000000000000000, 1.000000000000000000 ) ) ;
#14741=CIRCLE ( 'NONE', #24334, 3.500000000000003109 ) ;
#14748=AXIS2_PLACEMENT_3D ( 'NONE', #21236, #24237, #16000 ) ;
#14754=DIRECTION ( 'NONE',  ( 1.000000000000000000, -9.251858538542971828E-16, 0.000000000000000000 ) ) ;
#14782=VECTOR ( 'NONE', #21404, 999.9999999999998863 ) ;
#14795=CIRCLE ( 'NONE', #35188, 30.00000000000000000 ) ;
#14810=DIRECTION ( 'NONE',  ( -1.000000000000000000, 0.000000000000000000, 0.000000000000000000 ) ) ;
#14820=FACE_OUTER_BOUND ( 'NONE', #20866, .T. ) ;
#14830=CARTESIAN_POINT ( 'NONE',  ( -4.242640687119340726, -4.242640687119236809, 32.50000000000000000 ) ) ;
#14835=PLANE ( 'NONE',  #9950 ) ;
#14881=ORIENTED_EDGE ( 'NONE', *, *, #8478, .T. ) ;
#14888=ORIENTED_EDGE ( 'NONE', *, *, #3019, .T. ) ;
#14895=FACE_OUTER_BOUND ( 'NONE', #27478, .T. ) ;
#14896=EDGE_LOOP ( 'NONE', ( #12710, #27184, #4828, #11750 ) ) ;
#14899=FACE_OUTER_BOUND ( 'NONE', #6277, .T. ) ;
#14908=CARTESIAN_POINT ( 'NONE',  ( -102.5304832720481869, 102.5304832720506596, 32.50000000000000000 ) ) ;
#14924=EDGE_LOOP ( 'NONE', ( #16642, #37034, #25494, #32474 ) ) ;
#14967=CYLINDRICAL_SURFACE ( 'NONE', #15923, 3.500000000000003109 ) ;
#14970=DIRECTION ( 'NONE',  ( 0.000000000000000000, 0.000000000000000000, 1.000000000000000000 ) ) ;
#14993=ORIENTED_EDGE ( 'NONE', *, *, #27050, .T. ) ;
#14996=ORIENTED_EDGE ( 'NONE', *, *, #5384, .F. ) ;
#15000=DIRECTION ( 'NONE',  ( -0.000000000000000000, -0.000000000000000000, 1.000000000000000000 ) ) ;
#15002=EDGE_LOOP ( 'NONE', ( #29274, #10779, #6712, #13247 ) ) ;
#15004=DIRECTION ( 'NONE',  ( 0.000000000000000000, 0.000000000000000000, -1.000000000000000000 ) ) ;
#15005=CARTESIAN_POINT ( 'NONE',  ( -145.0000000000000000, 6.000000000001517009, 32.55002500000000509 ) ) ;
#15009=CARTESIAN_POINT ( 'NONE',  ( 82.27241335952179213, 47.49999999999982236, 27.50000000000000000 ) ) ;
#15010=VERTEX_POINT ( 'NONE', #16837 ) ;
#15030=DIRECTION ( 'NONE',  ( 0.000000000000000000, 0.000000000000000000, 1.000000000000000000 ) ) ;
#15035=CARTESIAN_POINT ( 'NONE',  ( -105.2709382882094218, 37.58034962363107923, 32.50000000000000711 ) ) ;
#15059=ORIENTED_EDGE ( 'NONE', *, *, #17714, .F. ) ;
#15063=CARTESIAN_POINT ( 'NONE',  ( 102.5304832720496080, 102.5304832720492527, 32.55002500000000509 ) ) ;
#15065=CARTESIAN_POINT ( 'NONE',  ( -14.38831834687553446, -115.5694366505189237, 32.50000000000000000 ) ) ;
#15067=DIRECTION ( 'NONE',  ( 0.000000000000000000, 0.000000000000000000, 1.000000000000000000 ) ) ;
#15068=ORIENTED_EDGE ( 'NONE', *, *, #26296, .T. ) ;
#15070=ADVANCED_FACE ( 'NONE', ( #11735 ), #19648, .F. ) ;
#15073=ADVANCED_FACE ( 'NONE', ( #17200 ), #28256, .F. ) ;
#15077=CARTESIAN_POINT ( 'NONE',  ( 67.30619744049005249, 84.18124734178236679, 27.50000000000000000 ) ) ;
#15095=DIRECTION ( 'NONE',  ( 0.000000000000000000, 0.000000000000000000, 1.000000000000000000 ) ) ;
#15097=DIRECTION ( 'NONE',  ( 0.000000000000000000, 0.000000000000000000, 1.000000000000000000 ) ) ;
#15104=EDGE_CURVE ( 'NONE', #7234, #11585, #33895, .T. ) ;
#15115=ADVANCED_FACE ( 'NONE', ( #8568 ), #20002, .F. ) ;
#15131=CIRCLE ( 'NONE', #6752, 95.00000000000001421 ) ;
#15138=EDGE_LOOP ( 'NONE', ( #6024, #14433, #20591, #29805 ) ) ;
#15148=EDGE_CURVE ( 'NONE', #37066, #31753, #29533, .T. ) ;
#15163=EDGE_CURVE ( 'NONE', #1946, #29329, #32732, .T. ) ;
#15175=CARTESIAN_POINT ( 'NONE',  ( 102.6344459086133298, 62.23183214669949592, 32.50000000000000711 ) ) ;
#15179=VECTOR ( 'NONE', #11347, 1000.000000000000000 ) ;
#15204=AXIS2_PLACEMENT_3D ( 'NONE', #33034, #19177, #22335 ) ;
#15212=CARTESIAN_POINT ( 'NONE',  ( 102.5304832720488832, -102.5304832720499633, 32.50000000000000000 ) ) ;
#15232=ORIENTED_EDGE ( 'NONE', *, *, #33991, .T. ) ;
#15241=ORIENTED_EDGE ( 'NONE', *, *, #16507, .F. ) ;
#15276=CARTESIAN_POINT ( 'NONE',  ( -106.7731239591695669, -98.28784258492920856, 27.50000000000000000 ) ) ;
#15282=EDGE_CURVE ( 'NONE', #18446, #36954, #32901, .T. ) ;
#15290=DIRECTION ( 'NONE',  ( -0.000000000000000000, -0.000000000000000000, -1.000000000000000000 ) ) ;
#15297=CARTESIAN_POINT ( 'NONE',  ( 94.55012560584674475, -9.234378588654731601, 32.50000000000000000 ) ) ;
#15310=AXIS2_PLACEMENT_3D ( 'NONE', #13066, #22252, #33119 ) ;
#15348=ORIENTED_EDGE ( 'NONE', *, *, #20207, .T. ) ;
#15360=DIRECTION ( 'NONE',  ( -0.000000000000000000, -0.000000000000000000, -1.000000000000000000 ) ) ;
#15361=DIRECTION ( 'NONE',  ( 1.000000000000000000, 0.000000000000000000, 0.000000000000000000 ) ) ;
#15362=EDGE_CURVE ( 'NONE', #11631, #17956, #13763, .T. ) ;
#15363=ORIENTED_EDGE ( 'NONE', *, *, #13498, .T. ) ;
#15374=DIRECTION ( 'NONE',  ( -1.000000000000000000, 0.000000000000000000, 0.000000000000000000 ) ) ;
#15377=EDGE_CURVE ( 'NONE', #14541, #8770, #22228, .T. ) ;
#15388=AXIS2_PLACEMENT_3D ( 'NONE', #12478, #26927, #13041 ) ;
#15390=AXIS2_PLACEMENT_3D ( 'NONE', #1308, #4496, #12921 ) ;
#15405=ORIENTED_EDGE ( 'NONE', *, *, #27520, .T. ) ;
#15411=LINE ( 'NONE', #1164, #14782 ) ;
#15430=AXIS2_PLACEMENT_3D ( 'NONE', #30040, #3794, #4361 ) ;
#15432=DIRECTION ( 'NONE',  ( -0.000000000000000000, -0.000000000000000000, -1.000000000000000000 ) ) ;
#15481=ORIENTED_EDGE ( 'NONE', *, *, #8613, .T. ) ;
#15509=CYLINDRICAL_SURFACE ( 'NONE', #1641, 150.0000000000000284 ) ;
#15514=ORIENTED_EDGE ( 'NONE', *, *, #24453, .T. ) ;
#15518=AXIS2_PLACEMENT_3D ( 'NONE', #25012, #5495, #10756 ) ;
#15600=DIRECTION ( 'NONE',  ( 1.000000000000000000, 0.000000000000000000, 0.000000000000000000 ) ) ;
#15619=ORIENTED_EDGE ( 'NONE', *, *, #3035, .F. ) ;
#15626=VERTEX_POINT ( 'NONE', #641 ) ;
#15634=EDGE_LOOP ( 'NONE', ( #15405, #5356, #20989, #7953 ) ) ;
#15636=CARTESIAN_POINT ( 'NONE',  ( -40.99999999999999289, -103.4105893997321743, 32.50000000000000000 ) ) ;
#15668=CARTESIAN_POINT ( 'NONE',  ( 108.3061974404898820, 19.22934205794938478, 32.50000000000000000 ) ) ;
#15682=ORIENTED_EDGE ( 'NONE', *, *, #2366, .F. ) ;
#15690=DIRECTION ( 'NONE',  ( 1.000000000000000000, 0.000000000000000000, 0.000000000000000000 ) ) ;
#15701=LINE ( 'NONE', #30516, #25987 ) ;
#15733=DIRECTION ( 'NONE',  ( 0.000000000000000000, 0.000000000000000000, 1.000000000000000000 ) ) ;
#15735=LINE ( 'NONE', #24000, #1215 ) ;
#15759=CARTESIAN_POINT ( 'NONE',  ( -104.8061974404896262, 19.22934205795090534, 32.50000000000000000 ) ) ;
#15772=AXIS2_PLACEMENT_3D ( 'NONE', #14408, #19849, #22295 ) ;
#15773=ORIENTED_EDGE ( 'NONE', *, *, #36790, .F. ) ;
#15777=CARTESIAN_POINT ( 'NONE',  ( 106.7731239591688848, 98.28784258492994752, 27.50000000000000000 ) ) ;
#15826=ADVANCED_FACE ( 'NONE', ( #36246 ), #5490, .F. ) ;
#15894=AXIS2_PLACEMENT_3D ( 'NONE', #10381, #33258, #3070 ) ;
#15906=AXIS2_PLACEMENT_3D ( 'NONE', #10415, #28225, #2537 ) ;
#15917=VECTOR ( 'NONE', #19928, 1000.000000000000000 ) ;
#15918=DIRECTION ( 'NONE',  ( 1.000000000000000000, 0.000000000000000000, 0.000000000000000000 ) ) ;
#15923=AXIS2_PLACEMENT_3D ( 'NONE', #3535, #35021, #31648 ) ;
#15955=VECTOR ( 'NONE', #11101, 1000.000000000000000 ) ;
#15968=CARTESIAN_POINT ( 'NONE',  ( 51.68138994340220904, 113.8157894736842053, 32.50000000000000000 ) ) ;
#15987=ORIENTED_EDGE ( 'NONE', *, *, #25538, .T. ) ;
#16000=DIRECTION ( 'NONE',  ( 1.000000000000000000, 0.000000000000000000, 0.000000000000000000 ) ) ;
#16012=DIRECTION ( 'NONE',  ( -0.000000000000000000, -0.000000000000000000, 1.000000000000000000 ) ) ;
#16015=CARTESIAN_POINT ( 'NONE',  ( 139.0000000000000284, -5.056524707326808249E-13, 32.55002500000000509 ) ) ;
#16031=CARTESIAN_POINT ( 'NONE',  ( -40.99999999999999289, 103.4105893997321743, 32.50000000000000000 ) ) ;
#16070=ORIENTED_EDGE ( 'NONE', *, *, #6812, .F. ) ;
#16095=AXIS2_PLACEMENT_3D ( 'NONE', #3659, #29146, #20700 ) ;
#16096=VERTEX_POINT ( 'NONE', #8426 ) ;
#16138=CARTESIAN_POINT ( 'NONE',  ( -5.999999999999998224, -145.0000000000000568, 32.50000000000000000 ) ) ;
#16154=ADVANCED_FACE ( 'NONE', ( #5433 ), #14028, .T. ) ;
#16163=ORIENTED_EDGE ( 'NONE', *, *, #36253, .T. ) ;
#16182=CARTESIAN_POINT ( 'NONE',  ( -39.27785635698568711, -86.50000000000001421, 27.50000000000000000 ) ) ;
#16196=ADVANCED_FACE ( 'NONE', ( #11228 ), #22675, .F. ) ;
#16209=DIRECTION ( 'NONE',  ( -0.000000000000000000, -0.000000000000000000, 1.000000000000000000 ) ) ;
#16214=CARTESIAN_POINT ( 'NONE',  ( -94.55012560584690107, -9.234378588653415321, 32.50000000000000000 ) ) ;
#16222=CARTESIAN_POINT ( 'NONE',  ( 39.27785635698568711, 86.50000000000001421, 27.50000000000000000 ) ) ;
#16225=ORIENTED_EDGE ( 'NONE', *, *, #10544, .T. ) ;
#16252=FACE_OUTER_BOUND ( 'NONE', #9512, .T. ) ;
#16253=ORIENTED_EDGE ( 'NONE', *, *, #22651, .T. ) ;
#16254=CARTESIAN_POINT ( 'NONE',  ( 0.000000000000000000, 0.000000000000000000, 27.50000000000000000 ) ) ;
#16267=CARTESIAN_POINT ( 'NONE',  ( -107.2724133595221190, -47.49999999999924682, 32.50002500000000083 ) ) ;
#16269=CARTESIAN_POINT ( 'NONE',  ( -103.8783455066836297, 60.08523189856654056, 32.50000000000000000 ) ) ;
#16273=CARTESIAN_POINT ( 'NONE',  ( -39.27785635698568711, 86.50000000000001421, 32.50000000000000000 ) ) ;
#16275=CARTESIAN_POINT ( 'NONE',  ( -82.27241335952113843, 47.50000000000096634, 27.50000000000000000 ) ) ;
#16289=CYLINDRICAL_SURFACE ( 'NONE', #26298, 3.499999999999996003 ) ;
#16292=LINE ( 'NONE', #30342, #20268 ) ;
#16293=CARTESIAN_POINT ( 'NONE',  ( -102.3448362992174623, 32.57931213457970188, 32.50000000000000000 ) ) ;
#16299=CARTESIAN_POINT ( 'NONE',  ( -74.30619744049063513, -84.18124734178186941, 27.50000000000000000 ) ) ;
#16309=CARTESIAN_POINT ( 'NONE',  ( 74.30619744049005249, 84.18124734178236679, 27.50000000000000000 ) ) ;
#16311=VERTEX_POINT ( 'NONE', #26695 ) ;
#16314=LINE ( 'NONE', #27730, #17618 ) ;
#16328=( LENGTH_UNIT ( ) NAMED_UNIT ( * ) SI_UNIT ( .MILLI., .METRE. ) );
#16339=DIRECTION ( 'NONE',  ( 3.491481338843133750E-15, 1.000000000000000000, -0.000000000000000000 ) ) ;
#16355=CARTESIAN_POINT ( 'NONE',  ( -77.93343913441745485, -72.12058696850748163, 27.50000000000000000 ) ) ;
#16362=LINE ( 'NONE', #16553, #17769 ) ;
#16373=LINE ( 'NONE', #16015, #29443 ) ;
#16376=DIRECTION ( 'NONE',  ( 0.000000000000000000, 0.000000000000000000, 1.000000000000000000 ) ) ;
#16380=AXIS2_PLACEMENT_3D ( 'NONE', #1787, #27646, #4795 ) ;
#16390=CARTESIAN_POINT ( 'NONE',  ( 40.99999999999999289, 103.4105893997321743, 32.50000000000000000 ) ) ;
#16402=DIRECTION ( 'NONE',  ( -0.000000000000000000, -0.000000000000000000, 1.000000000000000000 ) ) ;
#16406=DIRECTION ( 'NONE',  ( 0.000000000000000000, 0.000000000000000000, 1.000000000000000000 ) ) ;
#16414=DIRECTION ( 'NONE',  ( -0.7071067811865388020, 0.7071067811865563435, 0.000000000000000000 ) ) ;
#16416=CARTESIAN_POINT ( 'NONE',  ( 6.497954182785949224E-14, 5.999999999999947597, 32.50000000000000000 ) ) ;
#16421=CYLINDRICAL_SURFACE ( 'NONE', #36513, 3.500000000000003109 ) ;
#16429=PLANE ( 'NONE',  #8196 ) ;
#16462=CARTESIAN_POINT ( 'NONE',  ( 108.3061974404897825, -19.22934205795014151, 32.50000000000000000 ) ) ;
#16463=DIRECTION ( 'NONE',  ( -0.000000000000000000, -0.000000000000000000, -1.000000000000000000 ) ) ;
#16473=CARTESIAN_POINT ( 'NONE',  ( 6.123233995736731770E-16, -145.0000000000000568, 32.55002500000000509 ) ) ;
#16474=CARTESIAN_POINT ( 'NONE',  ( -39.27785635698568711, 86.50000000000001421, 27.50000000000000000 ) ) ;
#16478=CARTESIAN_POINT ( 'NONE',  ( 80.47895202573684514, -72.44487385379852640, 32.50000000000000000 ) ) ;
#16487=PRESENTATION_STYLE_ASSIGNMENT (( #33378 ) ) ;
#16494=VECTOR ( 'NONE', #27663, 1000.000000000000000 ) ;
#16498=ORIENTED_EDGE ( 'NONE', *, *, #4175, .T. ) ;
#16507=EDGE_CURVE ( 'NONE', #17078, #18795, #19109, .T. ) ;
#16533=CIRCLE ( 'NONE', #24918, 6.000000000000005329 ) ;
#16535=ORIENTED_EDGE ( 'NONE', *, *, #10453, .T. ) ;
#16538=CIRCLE ( 'NONE', #13556, 150.0000000000000284 ) ;
#16539=EDGE_CURVE ( 'NONE', #17144, #37066, #3062, .T. ) ;
#16540=DIRECTION ( 'NONE',  ( 0.000000000000000000, 0.000000000000000000, 1.000000000000000000 ) ) ;
#16547=VECTOR ( 'NONE', #35291, 1000.000000000000000 ) ;
#16553=CARTESIAN_POINT ( 'NONE',  ( 4.242640687119251020, -4.242640687119268783, 32.50000000000000000 ) ) ;
#16559=ORIENTED_EDGE ( 'NONE', *, *, #6430, .F. ) ;
#16561=LINE ( 'NONE', #19368, #34105 ) ;
#16580=DIRECTION ( 'NONE',  ( 1.000000000000000000, 0.000000000000000000, 0.000000000000000000 ) ) ;
#16581=DIRECTION ( 'NONE',  ( 0.000000000000000000, 0.000000000000000000, 1.000000000000000000 ) ) ;
#16596=AXIS2_PLACEMENT_3D ( 'NONE', #2658, #11467, #25545 ) ;
#16597=CARTESIAN_POINT ( 'NONE',  ( 21.64608276454480063, -107.6288746094956537, 32.49999999999999289 ) ) ;
#16600=AXIS2_PLACEMENT_3D ( 'NONE', #24011, #35458, #27366 ) ;
#16622=VERTEX_POINT ( 'NONE', #22364 ) ;
#16624=EDGE_LOOP ( 'NONE', ( #29351, #7138, #7650, #35850 ) ) ;
#16642=ORIENTED_EDGE ( 'NONE', *, *, #3208, .F. ) ;
#16688=EDGE_CURVE ( 'NONE', #36954, #18446, #11900, .T. ) ;
#16702=CIRCLE ( 'NONE', #521, 6.000000000000005329 ) ;
#16723=ORIENTED_EDGE ( 'NONE', *, *, #17382, .T. ) ;
#16724=CARTESIAN_POINT ( 'NONE',  ( 34.00000000000000000, -103.4105893997321743, 32.50000000000000000 ) ) ;
#16732=ORIENTED_EDGE ( 'NONE', *, *, #6450, .F. ) ;
#16741=EDGE_LOOP ( 'NONE', ( #22508, #10731, #16989, #2203 ) ) ;
#16751=VERTEX_POINT ( 'NONE', #32071 ) ;
#16760=LINE ( 'NONE', #22005, #25268 ) ;
#16763=ORIENTED_EDGE ( 'NONE', *, *, #33907, .T. ) ;
#16780=ORIENTED_EDGE ( 'NONE', *, *, #13392, .F. ) ;
#16792=CARTESIAN_POINT ( 'NONE',  ( 18.19094855014379064, -112.1612271170976953, 32.50000000000000000 ) ) ;
#16806=EDGE_CURVE ( 'NONE', #1952, #30663, #20126, .T. ) ;
#16809=ORIENTED_EDGE ( 'NONE', *, *, #13309, .T. ) ;
#16811=DIRECTION ( 'NONE',  ( 0.000000000000000000, 0.000000000000000000, 1.000000000000000000 ) ) ;
#16830=VERTEX_POINT ( 'NONE', #5026 ) ;
#16834=DIRECTION ( 'NONE',  ( 1.000000000000000000, 0.000000000000000000, 0.000000000000000000 ) ) ;
#16837=CARTESIAN_POINT ( 'NONE',  ( -110.2237710830543733, -101.7384897088139724, 27.50000000000000000 ) ) ;
#16843=AXIS2_PLACEMENT_3D ( 'NONE', #4446, #9524, #23773 ) ;
#16857=CARTESIAN_POINT ( 'NONE',  ( -90.52724777280822366, -71.16956570548431671, 32.50000000000000000 ) ) ;
#16858=VECTOR ( 'NONE', #8048, 1000.000000000000000 ) ;
#16867=CARTESIAN_POINT ( 'NONE',  ( -102.5304832720503185, -102.5304832720485280, 32.50000000000000000 ) ) ;
#16882=VERTEX_POINT ( 'NONE', #19660 ) ;
#16884=ORIENTED_EDGE ( 'NONE', *, *, #1403, .T. ) ;
#16887=FACE_OUTER_BOUND ( 'NONE', #12971, .T. ) ;
#16892=VERTEX_POINT ( 'NONE', #22282 ) ;
#16894=CARTESIAN_POINT ( 'NONE',  ( -145.0000000000000000, 6.000000000001517009, 27.50000000000000000 ) ) ;
#16904=DIRECTION ( 'NONE',  ( -0.000000000000000000, -0.000000000000000000, 1.000000000000000000 ) ) ;
#16906=DIRECTION ( 'NONE',  ( 1.000000000000000000, 0.000000000000000000, 0.000000000000000000 ) ) ;
#16908=ORIENTED_EDGE ( 'NONE', *, *, #711, .T. ) ;
#16930=VECTOR ( 'NONE', #29516, 1000.000000000000000 ) ;
#16937=CARTESIAN_POINT ( 'NONE',  ( -23.49187026334539041, 103.5527527874234863, 27.49999400000000094 ) ) ;
#16939=DIRECTION ( 'NONE',  ( -0.000000000000000000, 0.000000000000000000, -1.000000000000000000 ) ) ;
#16947=ORIENTED_EDGE ( 'NONE', *, *, #21513, .T. ) ;
#16984=DIRECTION ( 'NONE',  ( 1.000000000000000000, 0.000000000000000000, -0.000000000000000000 ) ) ;
#16989=ORIENTED_EDGE ( 'NONE', *, *, #33993, .F. ) ;
#17000=ORIENTED_EDGE ( 'NONE', *, *, #7610, .F. ) ;
#17025=CARTESIAN_POINT ( 'NONE',  ( 79.20390285583188472, -72.31905506802638683, 32.50000000000002132 ) ) ;
#17043=ORIENTED_EDGE ( 'NONE', *, *, #2006, .F. ) ;
#17067=DIRECTION ( 'NONE',  ( 1.000000000000000000, 0.000000000000000000, 0.000000000000000000 ) ) ;
#17070=MECHANICAL_DESIGN_GEOMETRIC_PRESENTATION_REPRESENTATION('',(#25451),#21865);
#17078=VERTEX_POINT ( 'NONE', #694 ) ;
#17085=APPLICATION_CONTEXT ( 'automotive_design' ) ;
#17086=CARTESIAN_POINT ( 'NONE',  ( -74.30619744049063513, -84.18124734178186941, 32.50000000000000000 ) ) ;
#17093=CIRCLE ( 'NONE', #11090, 95.00000000000001421 ) ;
#17098=AXIS2_PLACEMENT_3D ( 'NONE', #9663, #29515, #34976 ) ;
#17117=FACE_OUTER_BOUND ( 'NONE', #16624, .T. ) ;
#17119=FACE_OUTER_BOUND ( 'NONE', #14896, .T. ) ;
#17120=CARTESIAN_POINT ( 'NONE',  ( -39.27785635698568711, 86.50000000000001421, 27.50000000000000000 ) ) ;
#17121=CARTESIAN_POINT ( 'NONE',  ( -12.25360682529215772, 116.9391560352561896, 27.49998800000000188 ) ) ;
#17129=DIRECTION ( 'NONE',  ( 1.000000000000000000, 0.000000000000000000, 0.000000000000000000 ) ) ;
#17144=VERTEX_POINT ( 'NONE', #29380 ) ;
#17170=ORIENTED_EDGE ( 'NONE', *, *, #21716, .F. ) ;
#17174=DIRECTION ( 'NONE',  ( -0.000000000000000000, -0.000000000000000000, 1.000000000000000000 ) ) ;
#17181=CIRCLE ( 'NONE', #35732, 5.999999999999999112 ) ;
#17187=AXIS2_PLACEMENT_3D ( 'NONE', #1604, #30098, #7607 ) ;
#17189=EDGE_LOOP ( 'NONE', ( #27843, #11818 ) ) ;
#17192=LINE ( 'NONE', #14548, #6929 ) ;
#17200=FACE_OUTER_BOUND ( 'NONE', #15634, .T. ) ;
#17211=CARTESIAN_POINT ( 'NONE',  ( -110.2237710830522559, 101.7384897088162745, 32.55002500000000509 ) ) ;
#17212=VERTEX_POINT ( 'NONE', #35215 ) ;
#17230=CARTESIAN_POINT ( 'NONE',  ( 107.1113102691238907, -50.40388046061509897, 32.50000000000000000 ) ) ;
#17232=CARTESIAN_POINT ( 'NONE',  ( 72.72667006429044534, -101.6652913307183610, 27.50000000000000000 ) ) ;
#17235=ORIENTED_EDGE ( 'NONE', *, *, #6450, .T. ) ;
#17247=ORIENTED_EDGE ( 'NONE', *, *, #7907, .F. ) ;
#17252=SURFACE_STYLE_USAGE ( .BOTH. , #13870 ) ;
#17259=AXIS2_PLACEMENT_3D ( 'NONE', #12189, #23659, #12587 ) ;
#17292=CARTESIAN_POINT ( 'NONE',  ( 108.3061974404897825, -19.22934205795014151, 32.50000000000000000 ) ) ;
#17299=CIRCLE ( 'NONE', #20875, 3.500000000000003109 ) ;
#17307=DIRECTION ( 'NONE',  ( 1.000000000000000000, 0.000000000000000000, 0.000000000000000000 ) ) ;
#17319=LINE ( 'NONE', #14663, #35545 ) ;
#17330=CARTESIAN_POINT ( 'NONE',  ( -72.72667006429185221, -101.6652913307173662, 32.50000000000000000 ) ) ;
#17380=ORIENTED_EDGE ( 'NONE', *, *, #29349, .F. ) ;
#17382=EDGE_CURVE ( 'NONE', #36317, #1952, #10624, .T. ) ;
#17402=ORIENTED_EDGE ( 'NONE', *, *, #31222, .F. ) ;
#17403=AXIS2_PLACEMENT_3D ( 'NONE', #26660, #18786, #7531 ) ;
#17410=DIRECTION ( 'NONE',  ( 1.000000000000000000, 0.000000000000000000, 0.000000000000000000 ) ) ;
#17421=EDGE_LOOP ( 'NONE', ( #1624, #32103, #17900, #11697 ) ) ;
#17429=ORIENTED_EDGE ( 'NONE', *, *, #23389, .T. ) ;
#17431=ORIENTED_EDGE ( 'NONE', *, *, #27292, .T. ) ;
#17438=DIRECTION ( 'NONE',  ( 0.000000000000000000, 0.000000000000000000, 1.000000000000000000 ) ) ;
#17439=CARTESIAN_POINT ( 'NONE',  ( 0.000000000000000000, 0.000000000000000000, 32.50000000000000000 ) ) ;
#17461=CYLINDRICAL_SURFACE ( 'NONE', #36883, 30.00000000000000000 ) ;
#17464=VECTOR ( 'NONE', #23906, 1000.000000000000000 ) ;
#17465=EDGE_CURVE ( 'NONE', #27468, #27651, #14795, .T. ) ;
#17467=DIRECTION ( 'NONE',  ( 1.000000000000000000, -3.846960960290410782E-15, 0.000000000000000000 ) ) ;
#17471=DIRECTION ( 'NONE',  ( 0.000000000000000000, -0.000000000000000000, -1.000000000000000000 ) ) ;
#17472=ORIENTED_EDGE ( 'NONE', *, *, #11911, .F. ) ;
#17481=DIRECTION ( 'NONE',  ( -1.000000000000000000, 0.000000000000000000, 0.000000000000000000 ) ) ;
#17487=DIRECTION ( 'NONE',  ( -0.000000000000000000, -0.000000000000000000, -1.000000000000000000 ) ) ;
#17500=AXIS2_PLACEMENT_3D ( 'NONE', #2093, #16540, #30970 ) ;
#17507=EDGE_LOOP ( 'NONE', ( #17689, #10955, #20798, #14140 ) ) ;
#17510=AXIS2_PLACEMENT_3D ( 'NONE', #12149, #15004, #14810 ) ;
#17511=CARTESIAN_POINT ( 'NONE',  ( -72.72667006429185221, -101.6652913307173662, 32.50002500000000083 ) ) ;
#17521=DIRECTION ( 'NONE',  ( 0.000000000000000000, 0.000000000000000000, 1.000000000000000000 ) ) ;
#17530=CYLINDRICAL_SURFACE ( 'NONE', #12962, 3.500000000000003109 ) ;
#17563=VERTEX_POINT ( 'NONE', #32695 ) ;
#17565=ORIENTED_EDGE ( 'NONE', *, *, #261, .F. ) ;
#17568=DIRECTION ( 'NONE',  ( 0.000000000000000000, 0.000000000000000000, 1.000000000000000000 ) ) ;
#17606=CARTESIAN_POINT ( 'NONE',  ( 90.51346025932915040, 71.13874598957531248, 32.50000000000000711 ) ) ;
#17612=DIRECTION ( 'NONE',  ( 1.000000000000000000, 0.000000000000000000, 0.000000000000000000 ) ) ;
#17615=CIRCLE ( 'NONE', #22418, 3.499999999999996003 ) ;
#17618=VECTOR ( 'NONE', #7316, 1000.000000000000000 ) ;
#17627=FACE_BOUND ( 'NONE', #31087, .T. ) ;
#17633=EDGE_CURVE ( 'NONE', #8115, #8678, #29168, .T. ) ;
#17653=CARTESIAN_POINT ( 'NONE',  ( 37.50000000000000000, 103.4105893997321743, 32.50000000000000000 ) ) ;
#17655=CARTESIAN_POINT ( 'NONE',  ( 37.50000000000000000, 103.4105893997321743, 27.50000000000000000 ) ) ;
#17666=CARTESIAN_POINT ( 'NONE',  ( 145.0000000000000853, 5.999999999999493738, 32.55002500000000509 ) ) ;
#17685=EDGE_LOOP ( 'NONE', ( #20987, #18140 ) ) ;
#17687=EDGE_LOOP ( 'NONE', ( #36586, #5934 ) ) ;
#17689=ORIENTED_EDGE ( 'NONE', *, *, #18404, .F. ) ;
#17711=VECTOR ( 'NONE', #33130, 999.9999999999998863 ) ;
#17714=EDGE_CURVE ( 'NONE', #19610, #7234, #20184, .T. ) ;
#17717=CARTESIAN_POINT ( 'NONE',  ( 0.000000000000000000, 0.000000000000000000, 27.50000000000000000 ) ) ;
#17726=LINE ( 'NONE', #23936, #31419 ) ;
#17730=VERTEX_POINT ( 'NONE', #27248 ) ;
#17735=VECTOR ( 'NONE', #26761, 1000.000000000000000 ) ;
#17769=VECTOR ( 'NONE', #27982, 1000.000000000000114 ) ;
#17770=ORIENTED_EDGE ( 'NONE', *, *, #12027, .F. ) ;
#17774=PLANE ( 'NONE',  #12509 ) ;
#17776=CIRCLE ( 'NONE', #12986, 3.500000000000003109 ) ;
#17786=VERTEX_POINT ( 'NONE', #16214 ) ;
#17798=VERTEX_POINT ( 'NONE', #33641 ) ;
#17800=VECTOR ( 'NONE', #29474, 1000.000000000000000 ) ;
#17805=VECTOR ( 'NONE', #30067, 1000.000000000000000 ) ;
#17806=CARTESIAN_POINT ( 'NONE',  ( 105.1747985409462700, 37.32408539865060249, 32.49999999999999289 ) ) ;
#17807=DIRECTION ( 'NONE',  ( -1.000000000000000000, 1.082992363797667670E-14, 0.000000000000000000 ) ) ;
#17817=ADVANCED_FACE ( 'NONE', ( #6056 ), #11650, .F. ) ;
#17828=FACE_BOUND ( 'NONE', #17189, .T. ) ;
#17837=AXIS2_PLACEMENT_3D ( 'NONE', #30501, #1429, #18692 ) ;
#17843=ORIENTED_EDGE ( 'NONE', *, *, #1961, .T. ) ;
#17856=CARTESIAN_POINT ( 'NONE',  ( 0.000000000000000000, 0.000000000000000000, 32.50000000000000000 ) ) ;
#17885=DIRECTION ( 'NONE',  ( 0.000000000000000000, 0.000000000000000000, 1.000000000000000000 ) ) ;
#17886=ORIENTED_EDGE ( 'NONE', *, *, #36022, .T. ) ;
#17900=ORIENTED_EDGE ( 'NONE', *, *, #25538, .F. ) ;
#17921=ORIENTED_EDGE ( 'NONE', *, *, #32007, .T. ) ;
#17956=VERTEX_POINT ( 'NONE', #29088 ) ;
#17965=CARTESIAN_POINT ( 'NONE',  ( -107.2243249565953533, -49.31268038019268118, 32.50000000000000711 ) ) ;
#17969=ORIENTED_EDGE ( 'NONE', *, *, #21761, .F. ) ;
#17973=ORIENTED_EDGE ( 'NONE', *, *, #26296, .F. ) ;
#17994=CARTESIAN_POINT ( 'NONE',  ( 5.999999999999998224, 145.0000000000000568, 32.55002500000000509 ) ) ;
#17997=CARTESIAN_POINT ( 'NONE',  ( 96.68597835076329261, 67.93726906584150527, 32.49999999999999289 ) ) ;
#18018=FACE_BOUND ( 'NONE', #13081, .T. ) ;
#18060=CARTESIAN_POINT ( 'NONE',  ( -16.35104710633394376, -113.9564291516891927, 32.50000000000000000 ) ) ;
#18075=ORIENTED_EDGE ( 'NONE', *, *, #26763, .T. ) ;
#18080=ORIENTED_EDGE ( 'NONE', *, *, #5921, .F. ) ;
#18081=DIRECTION ( 'NONE',  ( 1.000000000000000000, 0.000000000000000000, 0.000000000000000000 ) ) ;
#18082=CARTESIAN_POINT ( 'NONE',  ( 39.27785635698568711, 86.50000000000001421, 27.50000000000000000 ) ) ;
#18087=ORIENTED_EDGE ( 'NONE', *, *, #28257, .T. ) ;
#18090=LINE ( 'NONE', #26910, #16930 ) ;
#18091=ORIENTED_EDGE ( 'NONE', *, *, #13643, .F. ) ;
#18102=DIRECTION ( 'NONE',  ( 0.7071067811865389130, -0.7071067811865561215, 0.000000000000000000 ) ) ;
#18129=LINE ( 'NONE', #35223, #17735 ) ;
#18140=ORIENTED_EDGE ( 'NONE', *, *, #24105, .T. ) ;
#18151=DIRECTION ( 'NONE',  ( 1.000000000000000000, 0.000000000000000000, 0.000000000000000000 ) ) ;
#18164=CARTESIAN_POINT ( 'NONE',  ( 0.000000000000000000, 0.000000000000000000, 32.50000000000000000 ) ) ;
#18165=DIRECTION ( 'NONE',  ( 1.000000000000000000, -3.554796214472773777E-16, 0.000000000000000000 ) ) ;
#18168=CARTESIAN_POINT ( 'NONE',  ( 98.28784258493033121, 106.7731239591685437, 27.50000000000000000 ) ) ;
#18169=CARTESIAN_POINT ( 'NONE',  ( -40.99999999999999289, -103.4105893997321743, 32.50000000000000000 ) ) ;
#18188=FACE_BOUND ( 'NONE', #33476, .T. ) ;
#18191=ORIENTED_EDGE ( 'NONE', *, *, #18273, .F. ) ;
#18210=CARTESIAN_POINT ( 'NONE',  ( -55.27226924886021919, 77.26562141134635908, 27.50000000000000000 ) ) ;
#18214=FACE_OUTER_BOUND ( 'NONE', #9200, .T. ) ;
#18219=VECTOR ( 'NONE', #24551, 1000.000000000000000 ) ;
#18220=ORIENTED_EDGE ( 'NONE', *, *, #26953, .T. ) ;
#18273=EDGE_CURVE ( 'NONE', #11585, #30663, #33089, .T. ) ;
#18292=CARTESIAN_POINT ( 'NONE',  ( -145.0000000000001137, -5.999999999998481215, 32.55002500000000509 ) ) ;
#18294=LINE ( 'NONE', #35564, #34969 ) ;
#18304=EDGE_CURVE ( 'NONE', #17144, #3455, #34303, .T. ) ;
#18308=CARTESIAN_POINT ( 'NONE',  ( 0.000000000000000000, 0.000000000000000000, 27.50000000000000000 ) ) ;
#18309=DIRECTION ( 'NONE',  ( -0.000000000000000000, -0.000000000000000000, -1.000000000000000000 ) ) ;
#18324=AXIS2_PLACEMENT_3D ( 'NONE', #25334, #5289, #27763 ) ;
#18340=EDGE_CURVE ( 'NONE', #32462, #25777, #21101, .T. ) ;
#18353=CIRCLE ( 'NONE', #29713, 3.499999999999996003 ) ;
#18366=DIRECTION ( 'NONE',  ( -0.000000000000000000, -0.000000000000000000, 1.000000000000000000 ) ) ;
#18383=VERTEX_POINT ( 'NONE', #18168 ) ;
#18395=DIRECTION ( 'NONE',  ( 0.000000000000000000, 0.000000000000000000, 1.000000000000000000 ) ) ;
#18404=EDGE_CURVE ( 'NONE', #16311, #20316, #19321, .T. ) ;
#18406=EDGE_CURVE ( 'NONE', #460, #30149, #28398, .T. ) ;
#18446=VERTEX_POINT ( 'NONE', #361 ) ;
#18454=ADVANCED_FACE ( 'NONE', ( #11796 ), #23255, .T. ) ;
#18456=ORIENTED_EDGE ( 'NONE', *, *, #17465, .T. ) ;
#18464=CIRCLE ( 'NONE', #1080, 30.00000000000000000 ) ;
#18469=CARTESIAN_POINT ( 'NONE',  ( 6.000000000000000000, -149.8799519615616305, 27.50000000000000000 ) ) ;
#18494=DIRECTION ( 'NONE',  ( -0.000000000000000000, 0.000000000000000000, 1.000000000000000000 ) ) ;
#18547=CIRCLE ( 'NONE', #32279, 30.00000000000000000 ) ;
#18556=CARTESIAN_POINT ( 'NONE',  ( -101.7384897088158766, -110.2237710830526112, 32.50000000000000000 ) ) ;
#18562=ORIENTED_EDGE ( 'NONE', *, *, #28888, .F. ) ;
#18571=VECTOR ( 'NONE', #24777, 1000.000000000000000 ) ;
#18575=DIRECTION ( 'NONE',  ( -1.000000000000000000, 0.000000000000000000, 0.000000000000000000 ) ) ;
#18582=VERTEX_POINT ( 'NONE', #32990 ) ;
#18590=UNCERTAINTY_MEASURE_WITH_UNIT (LENGTH_MEASURE( 1.000000000000000082E-05 ), #18939, 'distance_accuracy_value', 'NONE');
#18602=ORIENTED_EDGE ( 'NONE', *, *, #26497, .F. ) ;
#18605=CYLINDRICAL_SURFACE ( 'NONE', #27370, 5.999999999999999112 ) ;
#18617=ORIENTED_EDGE ( 'NONE', *, *, #2085, .T. ) ;
#18651=CARTESIAN_POINT ( 'NONE',  ( -107.2724133595211526, 47.50000000000096634, 32.50002500000000083 ) ) ;
#18674=EDGE_LOOP ( 'NONE', ( #23993, #15514, #26394, #9833 ) ) ;
#18692=DIRECTION ( 'NONE',  ( 1.000000000000000000, 0.000000000000000000, 0.000000000000000000 ) ) ;
#18707=ORIENTED_EDGE ( 'NONE', *, *, #25672, .T. ) ;
#18720=ADVANCED_FACE ( 'NONE', ( #28449 ), #2425, .F. ) ;
#18744=CYLINDRICAL_SURFACE ( 'NONE', #9040, 30.00000000000000000 ) ;
#18746=CARTESIAN_POINT ( 'NONE',  ( 102.2321609167755980, -32.43314223652354400, 32.50000000000000000 ) ) ;
#18762=ORIENTED_EDGE ( 'NONE', *, *, #25860, .F. ) ;
#18776=DIRECTION ( 'NONE',  ( -1.000000000000000000, 0.000000000000000000, 0.000000000000000000 ) ) ;
#18786=DIRECTION ( 'NONE',  ( 0.000000000000000000, 0.000000000000000000, 1.000000000000000000 ) ) ;
#18795=VERTEX_POINT ( 'NONE', #24474 ) ;
#18831=CARTESIAN_POINT ( 'NONE',  ( 96.53048327204888324, -102.5304832720499633, 32.50000000000000000 ) ) ;
#18854=DIRECTION ( 'NONE',  ( 1.000000000000000000, 0.000000000000000000, -0.000000000000000000 ) ) ;
#18914=CARTESIAN_POINT ( 'NONE',  ( -101.4252494179839488, 31.43181965331819683, 32.50001250000000397 ) ) ;
#18917=EDGE_LOOP ( 'NONE', ( #20533, #32079, #17973, #26121 ) ) ;
#18939=( LENGTH_UNIT ( ) NAMED_UNIT ( * ) SI_UNIT ( .MILLI., .METRE. ) );
#18942=DIRECTION ( 'NONE',  ( -0.000000000000000000, -0.000000000000000000, 1.000000000000000000 ) ) ;
#18945=UNCERTAINTY_MEASURE_WITH_UNIT (LENGTH_MEASURE( 1.000000000000000082E-05 ), #11779, 'distance_accuracy_value', 'NONE');
#18957=VECTOR ( 'NONE', #22193, 1000.000000000000000 ) ;
#19033=DIRECTION ( 'NONE',  ( -0.000000000000000000, -0.000000000000000000, 1.000000000000000000 ) ) ;
#19052=CARTESIAN_POINT ( 'NONE',  ( -124.4080600076932370, -12.15049814296501829, 32.50002500000000083 ) ) ;
#19055=AXIS2_PLACEMENT_3D ( 'NONE', #8911, #6652, #8717 ) ;
#19066=ADVANCED_FACE ( 'NONE', ( #61 ), #3431, .F. ) ;
#19086=ORIENTED_EDGE ( 'NONE', *, *, #13306, .F. ) ;
#19093=CARTESIAN_POINT ( 'NONE',  ( -107.0734680828344096, 50.67989423971658169, 32.50000000000000000 ) ) ;
#19098=ORIENTED_EDGE ( 'NONE', *, *, #26869, .T. ) ;
#19108=CIRCLE ( 'NONE', #19766, 6.000000000000005329 ) ;
#19109=CIRCLE ( 'NONE', #21473, 150.0000000000000284 ) ;
#19162=EDGE_CURVE ( 'NONE', #33879, #36954, #17319, .T. ) ;
#19168=EDGE_CURVE ( 'NONE', #22389, #13276, #31194, .T. ) ;
#19173=EDGE_LOOP ( 'NONE', ( #14602, #19875, #35034, #30811 ) ) ;
#19177=DIRECTION ( 'NONE',  ( -0.000000000000000000, -0.000000000000000000, 1.000000000000000000 ) ) ;
#19180=DIRECTION ( 'NONE',  ( -0.000000000000000000, -0.000000000000000000, 1.000000000000000000 ) ) ;
#19183=ORIENTED_EDGE ( 'NONE', *, *, #30935, .F. ) ;
#19187=CARTESIAN_POINT ( 'NONE',  ( 108.3061974404898820, 19.22934205794938478, 27.50000000000000000 ) ) ;
#19219=CARTESIAN_POINT ( 'NONE',  ( 21.38228493551344300, 108.2013385194334489, 27.49998799999999832 ) ) ;
#19223=LINE ( 'NONE', #16031, #22584 ) ;
#19226=ORIENTED_EDGE ( 'NONE', *, *, #14504, .T. ) ;
#19229=CARTESIAN_POINT ( 'NONE',  ( -70.80619744048887299, 84.18124734178336155, 32.50000000000000000 ) ) ;
#19240=CARTESIAN_POINT ( 'NONE',  ( 145.0000000000000853, 5.999999999999493738, 27.50000000000000000 ) ) ;
#19267=CARTESIAN_POINT ( 'NONE',  ( -105.5600153471429081, 56.84082786873509008, 32.50000000000000711 ) ) ;
#19284=ADVANCED_FACE ( 'NONE', ( #18214 ), #30408, .F. ) ;
#19321=CIRCLE ( 'NONE', #17510, 25.00000000000000000 ) ;
#19340=DIRECTION ( 'NONE',  ( 1.000000000000000000, 0.000000000000000000, 0.000000000000000000 ) ) ;
#19345=DIRECTION ( 'NONE',  ( -0.000000000000000000, -0.000000000000000000, 1.000000000000000000 ) ) ;
#19364=VECTOR ( 'NONE', #16939, 1000.000000000000000 ) ;
#19368=CARTESIAN_POINT ( 'NONE',  ( 6.000000000000000000, 0.000000000000000000, 32.50000000000000000 ) ) ;
#19394=EDGE_CURVE ( 'NONE', #19410, #13732, #2283, .T. ) ;
#19402=CARTESIAN_POINT ( 'NONE',  ( 23.49187040204899546, -103.5527524078059400, 32.50001250000000397 ) ) ;
#19410=VERTEX_POINT ( 'NONE', #23263 ) ;
#19422=DIRECTION ( 'NONE',  ( 0.000000000000000000, 0.000000000000000000, 1.000000000000000000 ) ) ;
#19429=CIRCLE ( 'NONE', #3256, 150.0000000000000284 ) ;
#19430=FACE_OUTER_BOUND ( 'NONE', #11349, .T. ) ;
#19441=VECTOR ( 'NONE', #27537, 1000.000000000000000 ) ;
#19446=LINE ( 'NONE', #25097, #2728 ) ;
#19447=ORIENTED_EDGE ( 'NONE', *, *, #29289, .F. ) ;
#19508=ORIENTED_EDGE ( 'NONE', *, *, #29584, .T. ) ;
#19509=ORIENTED_EDGE ( 'NONE', *, *, #16806, .T. ) ;
#19554=EDGE_LOOP ( 'NONE', ( #21654, #2820, #8267, #12688 ) ) ;
#19602=DIRECTION ( 'NONE',  ( 1.000000000000000000, 0.000000000000000000, 0.000000000000000000 ) ) ;
#19610=VERTEX_POINT ( 'NONE', #31850 ) ;
#19618=EDGE_CURVE ( 'NONE', #5071, #28766, #14610, .T. ) ;
#19624=EDGE_CURVE ( 'NONE', #7230, #20815, #4457, .T. ) ;
#19625=FACE_OUTER_BOUND ( 'NONE', #36364, .T. ) ;
#19641=CYLINDRICAL_SURFACE ( 'NONE', #26311, 95.00000000000001421 ) ;
#19647=AXIS2_PLACEMENT_3D ( 'NONE', #21002, #26260, #15374 ) ;
#19648=CYLINDRICAL_SURFACE ( 'NONE', #13122, 6.000000000000005329 ) ;
#19654=CARTESIAN_POINT ( 'NONE',  ( -149.8799519615615736, 6.000000000001555200, 32.50000000000000000 ) ) ;
#19660=CARTESIAN_POINT ( 'NONE',  ( 145.0000000000000853, 5.999999999999493738, 32.50000000000000000 ) ) ;
#19666=CIRCLE ( 'NONE', #1706, 3.500000000000003109 ) ;
#19668=FACE_OUTER_BOUND ( 'NONE', #10204, .T. ) ;
#19674=CARTESIAN_POINT ( 'NONE',  ( 84.91100539867409225, -72.42200467504753192, 32.49999999999999289 ) ) ;
#19700=EDGE_CURVE ( 'NONE', #2614, #114, #3248, .T. ) ;
#19703=AXIS2_PLACEMENT_3D ( 'NONE', #16867, #2440, #8980 ) ;
#19709=CARTESIAN_POINT ( 'NONE',  ( -108.3061974404900241, -19.22934205794863516, 27.50000000000000000 ) ) ;
#19741=DIRECTION ( 'NONE',  ( -0.000000000000000000, -0.000000000000000000, -1.000000000000000000 ) ) ;
#19761=DIRECTION ( 'NONE',  ( 1.000000000000000000, 0.000000000000000000, 0.000000000000000000 ) ) ;
#19762=AXIS2_PLACEMENT_3D ( 'NONE', #19052, #27652, #35738 ) ;
#19766=AXIS2_PLACEMENT_3D ( 'NONE', #9939, #941, #3756 ) ;
#19767=CARTESIAN_POINT ( 'NONE',  ( -18.28331348626797492, 112.2394285210100833, 27.49998800000000188 ) ) ;
#19778=ORIENTED_EDGE ( 'NONE', *, *, #26802, .T. ) ;
#19788=CARTESIAN_POINT ( 'NONE',  ( 12.20884028603261484, -116.8570725989752503, 32.50000000000000000 ) ) ;
#19792=ORIENTED_EDGE ( 'NONE', *, *, #26387, .T. ) ;
#19809=ORIENTED_EDGE ( 'NONE', *, *, #10328, .T. ) ;
#19812=DIRECTION ( 'NONE',  ( -0.000000000000000000, -0.000000000000000000, 1.000000000000000000 ) ) ;
#19817=CIRCLE ( 'NONE', #21608, 30.00000000000000000 ) ;
#19823=DIRECTION ( 'NONE',  ( 1.000000000000000000, 0.000000000000000000, 0.000000000000000000 ) ) ;
#19827=ORIENTED_EDGE ( 'NONE', *, *, #22911, .F. ) ;
#19843=ORIENTED_EDGE ( 'NONE', *, *, #34206, .F. ) ;
#19849=DIRECTION ( 'NONE',  ( 0.000000000000000000, 0.000000000000000000, 1.000000000000000000 ) ) ;
#19851=CARTESIAN_POINT ( 'NONE',  ( -104.1070924947364205, -59.68425981333875541, 32.50000000000000000 ) ) ;
#19854=DIRECTION ( 'NONE',  ( 1.000000000000000000, 0.000000000000000000, 0.000000000000000000 ) ) ;
#19856=VERTEX_POINT ( 'NONE', #21734 ) ;
#19862=ORIENTED_EDGE ( 'NONE', *, *, #36253, .F. ) ;
#19871=CARTESIAN_POINT ( 'NONE',  ( 110.2237710830529664, -101.7384897088154929, 27.50000000000000000 ) ) ;
#19872=ADVANCED_FACE ( 'NONE', ( #11567 ), #25847, .F. ) ;
#19875=ORIENTED_EDGE ( 'NONE', *, *, #27556, .T. ) ;
#19892=CARTESIAN_POINT ( 'NONE',  ( -37.50000000000000000, -103.4105893997321743, 32.50000000000000000 ) ) ;
#19896=CARTESIAN_POINT ( 'NONE',  ( 94.55012560584681580, 9.234378588654079678, 32.50000000000000000 ) ) ;
#19901=DIRECTION ( 'NONE',  ( 1.000000000000000000, 0.000000000000000000, 0.000000000000000000 ) ) ;
#19910=CIRCLE ( 'NONE', #2551, 3.500000000000003109 ) ;
#19912=CARTESIAN_POINT ( 'NONE',  ( -108.3061974404900241, -19.22934205794863516, 32.50000000000000000 ) ) ;
#19923=AXIS2_PLACEMENT_3D ( 'NONE', #8280, #17438, #36765 ) ;
#19928=DIRECTION ( 'NONE',  ( -0.000000000000000000, -0.000000000000000000, 1.000000000000000000 ) ) ;
#19937=FACE_OUTER_BOUND ( 'NONE', #963, .T. ) ;
#19944=DIRECTION ( 'NONE',  ( 1.000000000000000000, 0.000000000000000000, 0.000000000000000000 ) ) ;
#19961=ADVANCED_FACE ( 'NONE', ( #1809 ), #36115, .T. ) ;
#19972=CYLINDRICAL_SURFACE ( 'NONE', #31712, 30.00000000000000000 ) ;
#20002=PLANE ( 'NONE',  #12514 ) ;
#20015=EDGE_LOOP ( 'NONE', ( #11994, #26205, #4717, #9155 ) ) ;
#20050=EDGE_LOOP ( 'NONE', ( #935, #4599, #22266, #18562 ) ) ;
#20079=CARTESIAN_POINT ( 'NONE',  ( 0.000000000000000000, 0.000000000000000000, 27.50000000000000000 ) ) ;
#20081=ORIENTED_EDGE ( 'NONE', *, *, #17714, .T. ) ;
#20088=VECTOR ( 'NONE', #7174, 1000.000000000000000 ) ;
#20100=EDGE_CURVE ( 'NONE', #27793, #22736, #36813, .T. ) ;
#20126=CIRCLE ( 'NONE', #21923, 30.00000000000000000 ) ;
#20145=CARTESIAN_POINT ( 'NONE',  ( 145.0000000000000284, -6.000000000000504485, 27.50000000000000000 ) ) ;
#20150=AXIS2_PLACEMENT_3D ( 'NONE', #1262, #24076, #1012 ) ;
#20151=AXIS2_PLACEMENT_3D ( 'NONE', #31598, #19812, #34253 ) ;
#20153=DIRECTION ( 'NONE',  ( 0.000000000000000000, -0.000000000000000000, -1.000000000000000000 ) ) ;
#20161=CARTESIAN_POINT ( 'NONE',  ( 0.000000000000000000, 0.000000000000000000, 32.50000000000000000 ) ) ;
#20184=CIRCLE ( 'NONE', #20784, 30.00000000000000000 ) ;
#20188=ORIENTED_EDGE ( 'NONE', *, *, #33706, .T. ) ;
#20190=VECTOR ( 'NONE', #24445, 1000.000000000000000 ) ;
#20191=EDGE_CURVE ( 'NONE', #14464, #32620, #20340, .T. ) ;
#20207=EDGE_CURVE ( 'NONE', #25010, #16622, #3098, .T. ) ;
#20222=CARTESIAN_POINT ( 'NONE',  ( -98.28784258493107018, -106.7731239591678474, 32.55002500000000509 ) ) ;
#20225=AXIS2_PLACEMENT_3D ( 'NONE', #17653, #11481, #56 ) ;
#20229=ORIENTED_EDGE ( 'NONE', *, *, #6220, .T. ) ;
#20242=PRODUCT ( 'mounting backplate', 'mounting backplate', '', ( #1422 ) ) ;
#20262=DIRECTION ( 'NONE',  ( 0.7071067811865536790, 0.7071067811865414665, 0.000000000000000000 ) ) ;
#20266=CARTESIAN_POINT ( 'NONE',  ( 34.00000000000000000, 103.4105893997321743, 32.50000000000000000 ) ) ;
#20268=VECTOR ( 'NONE', #27706, 1000.000000000000000 ) ;
#20301=CARTESIAN_POINT ( 'NONE',  ( -94.55012560584668790, 9.234378588655390629, 32.50000000000000000 ) ) ;
#20315=VERTEX_POINT ( 'NONE', #35198 ) ;
#20316=VERTEX_POINT ( 'NONE', #30100 ) ;
#20340=LINE ( 'NONE', #13963, #13974 ) ;
#20354=VERTEX_POINT ( 'NONE', #15297 ) ;
#20366=EDGE_CURVE ( 'NONE', #31806, #27793, #18294, .T. ) ;
#20372=VERTEX_POINT ( 'NONE', #7059 ) ;
#20380=CARTESIAN_POINT ( 'NONE',  ( 0.000000000000000000, 0.000000000000000000, 32.50000000000000000 ) ) ;
#20393=DIRECTION ( 'NONE',  ( 1.000000000000000000, 0.000000000000000000, 0.000000000000000000 ) ) ;
#20398=DIRECTION ( 'NONE',  ( 3.554796214472773777E-16, 1.000000000000000000, -0.000000000000000000 ) ) ;
#20424=EDGE_LOOP ( 'NONE', ( #26990, #23606, #26876, #27371 ) ) ;
#20446=FACE_BOUND ( 'NONE', #29582, .T. ) ;
#20459=ORIENTED_EDGE ( 'NONE', *, *, #7100, .T. ) ;
#20504=FACE_OUTER_BOUND ( 'NONE', #36936, .T. ) ;
#20509=LINE ( 'NONE', #3827, #24267 ) ;
#20518=CARTESIAN_POINT ( 'NONE',  ( 101.4252494179806661, -31.43181965332042438, 32.50001250000000397 ) ) ;
#20526=VECTOR ( 'NONE', #4789, 1000.000000000000000 ) ;
#20533=ORIENTED_EDGE ( 'NONE', *, *, #12830, .F. ) ;
#20536=CARTESIAN_POINT ( 'NONE',  ( 70.80619744049005249, 84.18124734178236679, 32.50000000000000000 ) ) ;
#20546=LINE ( 'NONE', #511, #10752 ) ;
#20557=AXIS2_PLACEMENT_3D ( 'NONE', #33425, #27606, #7739 ) ;
#20562=LINE ( 'NONE', #3331, #21296 ) ;
#20574=ORIENTED_EDGE ( 'NONE', *, *, #15163, .F. ) ;
#20579=ORIENTED_EDGE ( 'NONE', *, *, #19618, .F. ) ;
#20591=ORIENTED_EDGE ( 'NONE', *, *, #5205, .T. ) ;
#20600=CARTESIAN_POINT ( 'NONE',  ( 95.09677333951634637, 69.00170213796093321, 32.49999999999999289 ) ) ;
#20611=AXIS2_PLACEMENT_3D ( 'NONE', #14076, #188, #3196 ) ;
#20635=AXIS2_PLACEMENT_3D ( 'NONE', #4396, #30454, #27806 ) ;
#20649=DIRECTION ( 'NONE',  ( 0.000000000000000000, 0.000000000000000000, 1.000000000000000000 ) ) ;
#20668=LINE ( 'NONE', #34936, #2861 ) ;
#20682=AXIS2_PLACEMENT_3D ( 'NONE', #3878, #26765, #1078 ) ;
#20689=CARTESIAN_POINT ( 'NONE',  ( 145.0000000000000568, -5.056524707326808249E-13, 27.50000000000000000 ) ) ;
#20700=DIRECTION ( 'NONE',  ( -1.000000000000000000, 0.000000000000000000, 0.000000000000000000 ) ) ;
#20701=DIRECTION ( 'NONE',  ( 1.000000000000000000, 0.000000000000000000, 0.000000000000000000 ) ) ;
#20704=DIRECTION ( 'NONE',  ( -0.000000000000000000, -0.000000000000000000, -1.000000000000000000 ) ) ;
#20707=DIRECTION ( 'NONE',  ( 1.000000000000000000, 0.000000000000000000, 0.000000000000000000 ) ) ;
#20719=CIRCLE ( 'NONE', #35701, 3.500000000000003109 ) ;
#20721=CIRCLE ( 'NONE', #33320, 6.000000000000005329 ) ;
#20733=DIRECTION ( 'NONE',  ( 0.000000000000000000, 0.000000000000000000, 1.000000000000000000 ) ) ;
#20749=EDGE_LOOP ( 'NONE', ( #33881, #22071, #29232, #15363 ) ) ;
#20784=AXIS2_PLACEMENT_3D ( 'NONE', #27452, #8126, #24467 ) ;
#20798=ORIENTED_EDGE ( 'NONE', *, *, #7587, .T. ) ;
#20803=DIRECTION ( 'NONE',  ( 0.000000000000000000, 0.000000000000000000, 1.000000000000000000 ) ) ;
#20815=VERTEX_POINT ( 'NONE', #1712 ) ;
#20817=EDGE_CURVE ( 'NONE', #20354, #1224, #3828, .T. ) ;
#20830=VECTOR ( 'NONE', #4532, 1000.000000000000000 ) ;
#20832=VERTEX_POINT ( 'NONE', #19871 ) ;
#20842=AXIS2_PLACEMENT_3D ( 'NONE', #36734, #25478, #31650 ) ;
#20850=DIRECTION ( 'NONE',  ( -0.7071067811865539010, -0.7071067811865411334, 0.000000000000000000 ) ) ;
#20866=EDGE_LOOP ( 'NONE', ( #3210, #33841, #32751, #35382 ) ) ;
#20872=VERTEX_POINT ( 'NONE', #10877 ) ;
#20875=AXIS2_PLACEMENT_3D ( 'NONE', #29816, #3588, #12565 ) ;
#20877=DIRECTION ( 'NONE',  ( -0.000000000000000000, -0.000000000000000000, -1.000000000000000000 ) ) ;
#20886=DIRECTION ( 'NONE',  ( -1.000000000000000000, 0.000000000000000000, 0.000000000000000000 ) ) ;
#20905=ORIENTED_EDGE ( 'NONE', *, *, #21513, .F. ) ;
#20913=FACE_OUTER_BOUND ( 'NONE', #9433, .T. ) ;
#20922=ORIENTED_EDGE ( 'NONE', *, *, #29399, .F. ) ;
#20927=DIRECTION ( 'NONE',  ( 1.000000000000000000, -3.846960960290410782E-15, 0.000000000000000000 ) ) ;
#20955=DIRECTION ( 'NONE',  ( 0.000000000000000000, 0.000000000000000000, 1.000000000000000000 ) ) ;
#20959=CARTESIAN_POINT ( 'NONE',  ( -23.49187026334539041, 103.5527527874234863, 27.49999400000000094 ) ) ;
#20969=ORIENTED_EDGE ( 'NONE', *, *, #22232, .F. ) ;
#20987=ORIENTED_EDGE ( 'NONE', *, *, #28216, .T. ) ;
#20989=ORIENTED_EDGE ( 'NONE', *, *, #13290, .F. ) ;
#20994=CARTESIAN_POINT ( 'NONE',  ( 102.2320902944790788, 32.43306441797120243, 32.50000000000000000 ) ) ;
#21002=CARTESIAN_POINT ( 'NONE',  ( 124.4080600076931375, 12.15049814296589226, 32.50002500000000083 ) ) ;
#21005=ORIENTED_EDGE ( 'NONE', *, *, #28591, .F. ) ;
#21029=DIRECTION ( 'NONE',  ( -0.000000000000000000, -0.000000000000000000, -1.000000000000000000 ) ) ;
#21089=DIRECTION ( 'NONE',  ( -1.000000000000000000, 1.082992363797667670E-14, 0.000000000000000000 ) ) ;
#21100=ADVANCED_FACE ( 'NONE', ( #23988 ), #21343, .F. ) ;
#21101=CIRCLE ( 'NONE', #27681, 95.00000000000001421 ) ;
#21105=ORIENTED_EDGE ( 'NONE', *, *, #2085, .F. ) ;
#21110=ORIENTED_EDGE ( 'NONE', *, *, #6528, .T. ) ;
#21121=CARTESIAN_POINT ( 'NONE',  ( 110.2237710830536770, 101.7384897088147397, 32.50000000000000000 ) ) ;
#21128=EDGE_CURVE ( 'NONE', #25525, #27555, #33347, .T. ) ;
#21137=ORIENTED_EDGE ( 'NONE', *, *, #28257, .F. ) ;
#21139=ORIENTED_EDGE ( 'NONE', *, *, #615, .T. ) ;
#21145=EDGE_CURVE ( 'NONE', #16311, #31164, #1661, .T. ) ;
#21166=DIRECTION ( 'NONE',  ( 1.000000000000000000, 0.000000000000000000, 0.000000000000000000 ) ) ;
#21167=CYLINDRICAL_SURFACE ( 'NONE', #31734, 3.499999999999996003 ) ;
#21170=CARTESIAN_POINT ( 'NONE',  ( 88.03899772796695800, 71.83443712190781127, 32.50000000000000000 ) ) ;
#21179=CARTESIAN_POINT ( 'NONE',  ( 2.094888803305880329E-14, 6.000000000000000000, 27.50000000000000000 ) ) ;
#21221=EDGE_LOOP ( 'NONE', ( #20922, #9911, #26482, #6205 ) ) ;
#21228=CARTESIAN_POINT ( 'NONE',  ( -23.49154088336464241, -103.5526315789473699, 27.50000000000000000 ) ) ;
#21231=ORIENTED_EDGE ( 'NONE', *, *, #11932, .T. ) ;
#21232=CYLINDRICAL_SURFACE ( 'NONE', #32866, 6.000000000000005329 ) ;
#21236=CARTESIAN_POINT ( 'NONE',  ( -70.80619744048887299, 84.18124734178336155, 32.50000000000000000 ) ) ;
#21245=EDGE_LOOP ( 'NONE', ( #18762, #25120, #2991, #17429 ) ) ;
#21255=FACE_OUTER_BOUND ( 'NONE', #10669, .T. ) ;
#21260=DIRECTION ( 'NONE',  ( -0.000000000000000000, 0.000000000000000000, -1.000000000000000000 ) ) ;
#21262=AXIS2_PLACEMENT_3D ( 'NONE', #35944, #32934, #24503 ) ;
#21280=DIRECTION ( 'NONE',  ( 1.000000000000000000, 0.000000000000000000, 0.000000000000000000 ) ) ;
#21284=FACE_BOUND ( 'NONE', #26870, .T. ) ;
#21296=VECTOR ( 'NONE', #8589, 1000.000000000000000 ) ;
#21302=CARTESIAN_POINT ( 'NONE',  ( -70.80619744048887299, 84.18124734178336155, 32.50000000000000000 ) ) ;
#21332=ORIENTED_EDGE ( 'NONE', *, *, #10453, .F. ) ;
#21343=PLANE ( 'NONE',  #36224 ) ;
#21344=AXIS2_PLACEMENT_3D ( 'NONE', #5588, #14721, #2427 ) ;
#21353=AXIS2_PLACEMENT_3D ( 'NONE', #21668, #9850, #6851 ) ;
#21378=CIRCLE ( 'NONE', #21344, 5.999999999999999112 ) ;
#21380=LINE ( 'NONE', #26825, #22940 ) ;
#21385=AXIS2_PLACEMENT_3D ( 'NONE', #8896, #30384, #36396 ) ;
#21401=CIRCLE ( 'NONE', #14225, 150.0000000000000284 ) ;
#21404=DIRECTION ( 'NONE',  ( -0.7071067811865388020, 0.7071067811865563435, 0.000000000000000000 ) ) ;
#21410=( GEOMETRIC_REPRESENTATION_CONTEXT ( 3 ) GLOBAL_UNCERTAINTY_ASSIGNED_CONTEXT ( ( #18945 ) ) GLOBAL_UNIT_ASSIGNED_CONTEXT ( ( #11779, #23041, #11247 ) ) REPRESENTATION_CONTEXT ( 'NONE', 'WORKASPACE' ) );
#21425=LINE ( 'NONE', #27039, #23550 ) ;
#21442=EDGE_CURVE ( 'NONE', #13349, #3694, #11653, .T. ) ;
#21472=ORIENTED_EDGE ( 'NONE', *, *, #15377, .T. ) ;
#21473=AXIS2_PLACEMENT_3D ( 'NONE', #25916, #11307, #17307 ) ;
#21482=EDGE_CURVE ( 'NONE', #24628, #35778, #23042, .T. ) ;
#21513=EDGE_CURVE ( 'NONE', #3560, #36161, #26196, .T. ) ;
#21520=CYLINDRICAL_SURFACE ( 'NONE', #22580, 25.00000000000000000 ) ;
#21522=CARTESIAN_POINT ( 'NONE',  ( -107.0107044000184402, 51.13684811647830486, 32.50000000000000000 ) ) ;
#21530=FACE_OUTER_BOUND ( 'NONE', #24562, .T. ) ;
#21555=DIRECTION ( 'NONE',  ( -0.7071067811865539010, -0.7071067811865411334, 0.000000000000000000 ) ) ;
#21559=CIRCLE ( 'NONE', #34150, 3.500000000000003109 ) ;
#21579=CARTESIAN_POINT ( 'NONE',  ( -34.00000000000000000, -103.4105893997321743, 32.50000000000000000 ) ) ;
#21593=EDGE_LOOP ( 'NONE', ( #21472, #12606, #26452, #19827 ) ) ;
#21608=AXIS2_PLACEMENT_3D ( 'NONE', #27910, #2235, #28822 ) ;
#21617=CARTESIAN_POINT ( 'NONE',  ( -106.0139510964988290, -39.63064057142699426, 32.49999999999999289 ) ) ;
#21647=CYLINDRICAL_SURFACE ( 'NONE', #7748, 6.000000000000005329 ) ;
#21654=ORIENTED_EDGE ( 'NONE', *, *, #13092, .F. ) ;
#21665=FACE_BOUND ( 'NONE', #24852, .T. ) ;
#21668=CARTESIAN_POINT ( 'NONE',  ( -82.27241335952113843, 47.50000000000096634, 32.50002500000000083 ) ) ;
#21671=ORIENTED_EDGE ( 'NONE', *, *, #615, .F. ) ;
#21672=DIRECTION ( 'NONE',  ( 0.7071067811865435759, -0.7071067811865514585, 0.000000000000000000 ) ) ;
#21699=LINE ( 'NONE', #27131, #17711 ) ;
#21716=EDGE_CURVE ( 'NONE', #31750, #11964, #33499, .T. ) ;
#21720=CARTESIAN_POINT ( 'NONE',  ( -106.2330357599457642, 40.32855561135241373, 32.50000000000000000 ) ) ;
#21722=ORIENTED_EDGE ( 'NONE', *, *, #6583, .F. ) ;
#21734=CARTESIAN_POINT ( 'NONE',  ( -149.8799519615616873, -5.999999999998430589, 27.50000000000000000 ) ) ;
#21739=ORIENTED_EDGE ( 'NONE', *, *, #24800, .F. ) ;
#21750=ORIENTED_EDGE ( 'NONE', *, *, #15282, .T. ) ;
#21761=EDGE_CURVE ( 'NONE', #32044, #16751, #25608, .T. ) ;
#21786=ORIENTED_EDGE ( 'NONE', *, *, #13456, .F. ) ;
#21790=EDGE_CURVE ( 'NONE', #36317, #7201, #3321, .T. ) ;
#21812=DIRECTION ( 'NONE',  ( 0.7071067811865435759, -0.7071067811865514585, 0.000000000000000000 ) ) ;
#21822=EDGE_CURVE ( 'NONE', #24921, #17786, #30272, .T. ) ;
#21840=FACE_BOUND ( 'NONE', #3700, .T. ) ;
#21843=ADVANCED_FACE ( 'NONE', ( #14899 ), #23151, .F. ) ;
#21846=VECTOR ( 'NONE', #35387, 1000.000000000000000 ) ;
#21863=LINE ( 'NONE', #13244, #31014 ) ;
#21865=( GEOMETRIC_REPRESENTATION_CONTEXT ( 3 ) GLOBAL_UNCERTAINTY_ASSIGNED_CONTEXT ( ( #18590 ) ) GLOBAL_UNIT_ASSIGNED_CONTEXT ( ( #18939, #30567, #33745 ) ) REPRESENTATION_CONTEXT ( 'NONE', 'WORKASPACE' ) );
#21867=EDGE_CURVE ( 'NONE', #1598, #19410, #22262, .T. ) ;
#21905=DIRECTION ( 'NONE',  ( 1.000000000000000000, 0.000000000000000000, 0.000000000000000000 ) ) ;
#21911=ORIENTED_EDGE ( 'NONE', *, *, #1391, .T. ) ;
#21915=CARTESIAN_POINT ( 'NONE',  ( -124.4080600076929954, 12.15049814296761888, 27.50000000000000000 ) ) ;
#21923=AXIS2_PLACEMENT_3D ( 'NONE', #2025, #34107, #13842 ) ;
#21926=CARTESIAN_POINT ( 'NONE',  ( -101.6270506563345606, -63.51409607572428229, 32.50000000000000711 ) ) ;
#21927=DIRECTION ( 'NONE',  ( 1.000000000000000000, 0.000000000000000000, 0.000000000000000000 ) ) ;
#21934=ADVANCED_FACE ( 'NONE', ( #29135 ), #5718, .F. ) ;
#21939=CARTESIAN_POINT ( 'NONE',  ( 0.000000000000000000, 0.000000000000000000, 27.50000000000000000 ) ) ;
#21947=CIRCLE ( 'NONE', #4583, 30.00000000000000000 ) ;
#21952=DIRECTION ( 'NONE',  ( 0.000000000000000000, 0.000000000000000000, 1.000000000000000000 ) ) ;
#22005=CARTESIAN_POINT ( 'NONE',  ( 111.8061974404898962, 19.22934205794938478, 32.50000000000000000 ) ) ;
#22041=FACE_BOUND ( 'NONE', #2734, .T. ) ;
#22044=CIRCLE ( 'NONE', #8259, 150.0000000000000284 ) ;
#22046=EDGE_CURVE ( 'NONE', #17563, #17956, #24457, .T. ) ;
#22054=ORIENTED_EDGE ( 'NONE', *, *, #13309, .F. ) ;
#22061=CARTESIAN_POINT ( 'NONE',  ( 124.4080600076931375, 12.15049814296589226, 27.50000000000000000 ) ) ;
#22071=ORIENTED_EDGE ( 'NONE', *, *, #2366, .T. ) ;
#22109=DIRECTION ( 'NONE',  ( -0.000000000000000000, -0.000000000000000000, -1.000000000000000000 ) ) ;
#22124=CARTESIAN_POINT ( 'NONE',  ( 107.2801987736736180, -45.32358462409808197, 32.50000000000000711 ) ) ;
#22138=DIRECTION ( 'NONE',  ( 1.000000000000000000, 0.000000000000000000, 0.000000000000000000 ) ) ;
#22141=EDGE_CURVE ( 'NONE', #28369, #7532, #16760, .T. ) ;
#22183=ORIENTED_EDGE ( 'NONE', *, *, #35808, .F. ) ;
#22193=DIRECTION ( 'NONE',  ( -0.000000000000000000, -0.000000000000000000, -1.000000000000000000 ) ) ;
#22211=DIRECTION ( 'NONE',  ( 1.000000000000000000, 0.000000000000000000, 0.000000000000000000 ) ) ;
#22228=LINE ( 'NONE', #1605, #35326 ) ;
#22231=DIRECTION ( 'NONE',  ( -0.000000000000000000, -0.000000000000000000, -1.000000000000000000 ) ) ;
#22232=EDGE_CURVE ( 'NONE', #1598, #27017, #16373, .T. ) ;
#22245=DIRECTION ( 'NONE',  ( 0.000000000000000000, 0.000000000000000000, 1.000000000000000000 ) ) ;
#22252=DIRECTION ( 'NONE',  ( -0.000000000000000000, -0.000000000000000000, 1.000000000000000000 ) ) ;
#22262=CIRCLE ( 'NONE', #13873, 6.000000000000005329 ) ;
#22264=EDGE_LOOP ( 'NONE', ( #10486, #20229, #21750, #10847 ) ) ;
#22266=ORIENTED_EDGE ( 'NONE', *, *, #28320, .T. ) ;
#22276=CARTESIAN_POINT ( 'NONE',  ( 37.50000000000000000, -103.4105893997321743, 32.50000000000000000 ) ) ;
#22282=CARTESIAN_POINT ( 'NONE',  ( 106.7731239591682026, -98.28784258493068648, 27.50000000000000000 ) ) ;
#22289=DIRECTION ( 'NONE',  ( -0.000000000000000000, -0.000000000000000000, 1.000000000000000000 ) ) ;
#22295=DIRECTION ( 'NONE',  ( 1.000000000000000000, 0.000000000000000000, 0.000000000000000000 ) ) ;
#22296=CARTESIAN_POINT ( 'NONE',  ( 102.6344492401623398, -62.23201224809161403, 32.50000000000000711 ) ) ;
#22297=CARTESIAN_POINT ( 'NONE',  ( -86.97174780077182277, -72.12318266404240319, 32.49999999999999289 ) ) ;
#22298=DIRECTION ( 'NONE',  ( -0.000000000000000000, -0.000000000000000000, 1.000000000000000000 ) ) ;
#22306=CARTESIAN_POINT ( 'NONE',  ( -39.27785635698568711, -86.50000000000001421, 27.50000000000000000 ) ) ;
#22329=DIRECTION ( 'NONE',  ( 0.000000000000000000, 0.000000000000000000, 1.000000000000000000 ) ) ;
#22335=DIRECTION ( 'NONE',  ( 1.000000000000000000, 0.000000000000000000, 0.000000000000000000 ) ) ;
#22337=VECTOR ( 'NONE', #21089, 1000.000000000000000 ) ;
#22346=ORIENTED_EDGE ( 'NONE', *, *, #8957, .T. ) ;
#22364=CARTESIAN_POINT ( 'NONE',  ( -101.7384897088158766, -110.2237710830526112, 27.50000000000000000 ) ) ;
#22389=VERTEX_POINT ( 'NONE', #6215 ) ;
#22391=CYLINDRICAL_SURFACE ( 'NONE', #35902, 3.500000000000003109 ) ;
#22403=AXIS2_PLACEMENT_3D ( 'NONE', #36031, #21952, #10321 ) ;
#22405=CARTESIAN_POINT ( 'NONE',  ( -124.4080600076929954, 12.15049814296761888, 32.50002500000000083 ) ) ;
#22418=AXIS2_PLACEMENT_3D ( 'NONE', #35619, #22245, #21166 ) ;
#22419=CYLINDRICAL_SURFACE ( 'NONE', #385, 3.500000000000003109 ) ;
#22423=ORIENTED_EDGE ( 'NONE', *, *, #14558, .T. ) ;
#22434=AXIS2_PLACEMENT_3D ( 'NONE', #22405, #27664, #1613 ) ;
#22455=AXIS2_PLACEMENT_3D ( 'NONE', #25833, #35001, #31437 ) ;
#22465=AXIS2_PLACEMENT_3D ( 'NONE', #26931, #30102, #21672 ) ;
#22468=CARTESIAN_POINT ( 'NONE',  ( -95.78732839747756600, -68.56887374850442995, 32.49999999999999289 ) ) ;
#22471=CARTESIAN_POINT ( 'NONE',  ( 4.242640687119251020, -4.242640687119268783, 27.50000000000000000 ) ) ;
#22476=EDGE_CURVE ( 'NONE', #14464, #27264, #30695, .T. ) ;
#22480=CARTESIAN_POINT ( 'NONE',  ( -40.99999999999999289, 103.4105893997321743, 27.50000000000000000 ) ) ;
#22492=ORIENTED_EDGE ( 'NONE', *, *, #15362, .F. ) ;
#22508=ORIENTED_EDGE ( 'NONE', *, *, #35808, .T. ) ;
#22528=CARTESIAN_POINT ( 'NONE',  ( -37.50000000000000000, 103.4105893997321743, 32.50000000000000000 ) ) ;
#22556=FACE_OUTER_BOUND ( 'NONE', #2118, .T. ) ;
#22568=FACE_OUTER_BOUND ( 'NONE', #36803, .T. ) ;
#22575=EDGE_LOOP ( 'NONE', ( #10727, #31253, #1767, #2495 ) ) ;
#22580=AXIS2_PLACEMENT_3D ( 'NONE', #1830, #24888, #32958 ) ;
#22583=EDGE_CURVE ( 'NONE', #10982, #7521, #31091, .T. ) ;
#22584=VECTOR ( 'NONE', #19033, 1000.000000000000000 ) ;
#22586=DIRECTION ( 'NONE',  ( -0.7071067811865487940, -0.7071067811865463515, 0.000000000000000000 ) ) ;
#22587=EDGE_LOOP ( 'NONE', ( #21005, #4036, #28928, #4412 ) ) ;
#22608=DIRECTION ( 'NONE',  ( -0.000000000000000000, -0.000000000000000000, 1.000000000000000000 ) ) ;
#22609=AXIS2_PLACEMENT_3D ( 'NONE', #6653, #3825, #35710 ) ;
#22612=DIRECTION ( 'NONE',  ( 1.000000000000000000, 0.000000000000000000, 0.000000000000000000 ) ) ;
#22630=DIRECTION ( 'NONE',  ( 0.000000000000000000, 0.000000000000000000, 1.000000000000000000 ) ) ;
#22634=DIRECTION ( 'NONE',  ( -0.000000000000000000, -0.000000000000000000, 1.000000000000000000 ) ) ;
#22651=EDGE_CURVE ( 'NONE', #25777, #27468, #25839, .T. ) ;
#22672=CARTESIAN_POINT ( 'NONE',  ( 106.9297252919371175, -51.67691575806412629, 32.50000000000000000 ) ) ;
#22673=CARTESIAN_POINT ( 'NONE',  ( -106.8619808665325337, -52.03941024792912629, 32.50000000000000000 ) ) ;
#22675=CYLINDRICAL_SURFACE ( 'NONE', #12429, 3.500000000000003109 ) ;
#22685=VERTEX_POINT ( 'NONE', #14009 ) ;
#22692=VERTEX_POINT ( 'NONE', #8024 ) ;
#22698=EDGE_LOOP ( 'NONE', ( #10688, #12904, #25522, #36650 ) ) ;
#22735=ORIENTED_EDGE ( 'NONE', *, *, #13444, .T. ) ;
#22736=VERTEX_POINT ( 'NONE', #23761 ) ;
#22737=VECTOR ( 'NONE', #15290, 1000.000000000000000 ) ;
#22740=LINE ( 'NONE', #8475, #35684 ) ;
#22751=ORIENTED_EDGE ( 'NONE', *, *, #8930, .T. ) ;
#22752=VERTEX_POINT ( 'NONE', #35214 ) ;
#22764=LINE ( 'NONE', #34205, #15917 ) ;
#22772=CARTESIAN_POINT ( 'NONE',  ( 37.50000000000000000, 103.4105893997321743, 32.50000000000000000 ) ) ;
#22773=VECTOR ( 'NONE', #4221, 1000.000000000000000 ) ;
#22797=ORIENTED_EDGE ( 'NONE', *, *, #11911, .T. ) ;
#22811=CARTESIAN_POINT ( 'NONE',  ( 0.000000000000000000, 0.000000000000000000, 32.50000000000000000 ) ) ;
#22812=ORIENTED_EDGE ( 'NONE', *, *, #13, .T. ) ;
#22825=CYLINDRICAL_SURFACE ( 'NONE', #9300, 3.500000000000003109 ) ;
#22838=DIRECTION ( 'NONE',  ( -0.000000000000000000, -0.000000000000000000, -1.000000000000000000 ) ) ;
#22851=EDGE_CURVE ( 'NONE', #114, #12647, #26557, .T. ) ;
#22855=FACE_OUTER_BOUND ( 'NONE', #28687, .T. ) ;
#22861=CARTESIAN_POINT ( 'NONE',  ( -39.27785635698568711, -86.50000000000001421, 32.50000000000000000 ) ) ;
#22880=VERTEX_POINT ( 'NONE', #21121 ) ;
#22882=VERTEX_POINT ( 'NONE', #9696 ) ;
#22911=EDGE_CURVE ( 'NONE', #14541, #20832, #21863, .T. ) ;
#22923=EDGE_CURVE ( 'NONE', #29025, #34519, #9477, .T. ) ;
#22940=VECTOR ( 'NONE', #9580, 1000.000000000000000 ) ;
#22970=VECTOR ( 'NONE', #8978, 1000.000000000000000 ) ;
#22973=DIRECTION ( 'NONE',  ( 1.000000000000000000, 0.000000000000000000, 0.000000000000000000 ) ) ;
#22979=DIRECTION ( 'NONE',  ( -0.000000000000000000, -0.000000000000000000, -1.000000000000000000 ) ) ;
#22990=CARTESIAN_POINT ( 'NONE',  ( -106.7731239591675205, 98.28784258493143966, 32.55002500000000509 ) ) ;
#22993=ORIENTED_EDGE ( 'NONE', *, *, #6361, .T. ) ;
#23007=FACE_OUTER_BOUND ( 'NONE', #20424, .T. ) ;
#23040=EDGE_LOOP ( 'NONE', ( #22346, #33953, #21137, #33727 ) ) ;
#23041=( NAMED_UNIT ( * ) PLANE_ANGLE_UNIT ( ) SI_UNIT ( $, .RADIAN. ) );
#23042=CIRCLE ( 'NONE', #22455, 150.0000000000000284 ) ;
#23057=DIRECTION ( 'NONE',  ( 1.000000000000000000, 0.000000000000000000, 0.000000000000000000 ) ) ;
#23068=CARTESIAN_POINT ( 'NONE',  ( 23.49154088336464952, 103.5526315789473699, 32.50000000000000000 ) ) ;
#23084=ORIENTED_EDGE ( 'NONE', *, *, #29292, .F. ) ;
#23087=ORIENTED_EDGE ( 'NONE', *, *, #32007, .F. ) ;
#23094=CARTESIAN_POINT ( 'NONE',  ( -124.4080600076929954, 12.15049814296761888, 32.50000000000000000 ) ) ;
#23106=CARTESIAN_POINT ( 'NONE',  ( 82.27241335952147949, -47.50000000000039790, 32.50002500000000083 ) ) ;
#23112=AXIS2_PLACEMENT_3D ( 'NONE', #2885, #14111, #19761 ) ;
#23116=CARTESIAN_POINT ( 'NONE',  ( 101.4252628994511980, 31.43180897937319784, 32.50001250000000397 ) ) ;
#23136=CARTESIAN_POINT ( 'NONE',  ( 8.109924056054151009, -118.6579847640609131, 32.49999999999999289 ) ) ;
#23151=CYLINDRICAL_SURFACE ( 'NONE', #1294, 6.000000000000005329 ) ;
#23171=ADVANCED_FACE ( 'NONE', ( #23711 ), #26348, .F. ) ;
#23196=DIRECTION ( 'NONE',  ( 0.000000000000000000, 0.000000000000000000, 1.000000000000000000 ) ) ;
#23228=LINE ( 'NONE', #31459, #22970 ) ;
#23234=EDGE_LOOP ( 'NONE', ( #1643, #24482, #22993, #3525 ) ) ;
#23255=CYLINDRICAL_SURFACE ( 'NONE', #1962, 150.0000000000000284 ) ;
#23263=CARTESIAN_POINT ( 'NONE',  ( 145.0000000000000284, -6.000000000000504485, 32.50000000000000000 ) ) ;
#23268=ORIENTED_EDGE ( 'NONE', *, *, #15104, .F. ) ;
#23269=ORIENTED_EDGE ( 'NONE', *, *, #35933, .F. ) ;
#23284=DIRECTION ( 'NONE',  ( -3.846960960290410782E-15, -1.000000000000000000, 0.000000000000000000 ) ) ;
#23285=ORIENTED_EDGE ( 'NONE', *, *, #14217, .T. ) ;
#23316=DIRECTION ( 'NONE',  ( 1.000000000000000000, 0.000000000000000000, 0.000000000000000000 ) ) ;
#23321=VERTEX_POINT ( 'NONE', #18469 ) ;
#23326=DIRECTION ( 'NONE',  ( -0.000000000000000000, -0.000000000000000000, -1.000000000000000000 ) ) ;
#23333=CARTESIAN_POINT ( 'NONE',  ( -23.49188638668713480, -103.5527587461262442, 32.50001250000000397 ) ) ;
#23345=VERTEX_POINT ( 'NONE', #18831 ) ;
#23346=CARTESIAN_POINT ( 'NONE',  ( 104.8061974404898820, 19.22934205794938478, 32.50000000000000000 ) ) ;
#23348=DIRECTION ( 'NONE',  ( 0.000000000000000000, 0.000000000000000000, 1.000000000000000000 ) ) ;
#23366=DIRECTION ( 'NONE',  ( 0.000000000000000000, 0.000000000000000000, 1.000000000000000000 ) ) ;
#23377=EDGE_CURVE ( 'NONE', #20832, #13259, #21401, .T. ) ;
#23387=EDGE_CURVE ( 'NONE', #2049, #20372, #10378, .T. ) ;
#23389=EDGE_CURVE ( 'NONE', #12717, #13311, #434, .T. ) ;
#23402=EDGE_CURVE ( 'NONE', #8483, #32886, #35528, .T. ) ;
#23414=EDGE_CURVE ( 'NONE', #27264, #23728, #32694, .T. ) ;
#23469=CARTESIAN_POINT ( 'NONE',  ( -101.7384897088135887, 110.2237710830547286, 32.55002500000000509 ) ) ;
#23492=EDGE_LOOP ( 'NONE', ( #16225, #8204, #7823, #5457 ) ) ;
#23516=LINE ( 'NONE', #14698, #4116 ) ;
#23532=ORIENTED_EDGE ( 'NONE', *, *, #5205, .F. ) ;
#23538=ORIENTED_EDGE ( 'NONE', *, *, #4175, .F. ) ;
#23550=VECTOR ( 'NONE', #1355, 1000.000000000000000 ) ;
#23578=DIRECTION ( 'NONE',  ( 0.7071067811865536790, 0.7071067811865414665, 0.000000000000000000 ) ) ;
#23580=ORIENTED_EDGE ( 'NONE', *, *, #14347, .F. ) ;
#23587=DIRECTION ( 'NONE',  ( -1.047444401652940007E-14, -1.000000000000000000, 0.000000000000000000 ) ) ;
#23600=EDGE_LOOP ( 'NONE', ( #3474, #31883 ) ) ;
#23601=ORIENTED_EDGE ( 'NONE', *, *, #13392, .T. ) ;
#23606=ORIENTED_EDGE ( 'NONE', *, *, #17382, .F. ) ;
#23614=CYLINDRICAL_SURFACE ( 'NONE', #5779, 30.00000000000000000 ) ;
#23632=DIRECTION ( 'NONE',  ( 1.000000000000000000, 0.000000000000000000, 0.000000000000000000 ) ) ;
#23636=FACE_BOUND ( 'NONE', #7459, .T. ) ;
#23644=CARTESIAN_POINT ( 'NONE',  ( 40.99999999999999289, 103.4105893997321743, 27.50000000000000000 ) ) ;
#23651=VERTEX_POINT ( 'NONE', #20301 ) ;
#23659=DIRECTION ( 'NONE',  ( 0.000000000000000000, 0.000000000000000000, 1.000000000000000000 ) ) ;
#23687=ADVANCED_FACE ( 'NONE', ( #17117 ), #14313, .F. ) ;
#23688=DIRECTION ( 'NONE',  ( 1.000000000000000000, 0.000000000000000000, 0.000000000000000000 ) ) ;
#23692=AXIS2_PLACEMENT_3D ( 'NONE', #11517, #90, #8534 ) ;
#23699=ORIENTED_EDGE ( 'NONE', *, *, #6122, .T. ) ;
#23705=EDGE_LOOP ( 'NONE', ( #26371, #17000, #15348, #13280 ) ) ;
#23711=FACE_OUTER_BOUND ( 'NONE', #18917, .T. ) ;
#23714=EDGE_CURVE ( 'NONE', #11964, #11432, #219, .T. ) ;
#23721=CYLINDRICAL_SURFACE ( 'NONE', #28107, 6.000000000000005329 ) ;
#23728=VERTEX_POINT ( 'NONE', #5876 ) ;
#23758=EDGE_CURVE ( 'NONE', #20354, #36154, #34613, .T. ) ;
#23761=CARTESIAN_POINT ( 'NONE',  ( 94.40806000769313755, 12.15049814296589226, 27.50000000000000000 ) ) ;
#23773=DIRECTION ( 'NONE',  ( 1.000000000000000000, 0.000000000000000000, 0.000000000000000000 ) ) ;
#23789=EDGE_CURVE ( 'NONE', #25631, #24583, #35109, .T. ) ;
#23790=CIRCLE ( 'NONE', #5833, 3.500000000000003109 ) ;
#23794=LINE ( 'NONE', #35246, #27214 ) ;
#23815=CARTESIAN_POINT ( 'NONE',  ( 98.70586713948475222, 66.35239263737575754, 32.49999999999999289 ) ) ;
#23816=DIRECTION ( 'NONE',  ( 1.000000000000000000, 0.000000000000000000, 0.000000000000000000 ) ) ;
#23820=FACE_OUTER_BOUND ( 'NONE', #13951, .T. ) ;
#23824=VERTEX_POINT ( 'NONE', #15777 ) ;
#23830=DIRECTION ( 'NONE',  ( 0.000000000000000000, 0.000000000000000000, 1.000000000000000000 ) ) ;
#23835=AXIS2_PLACEMENT_3D ( 'NONE', #3824, #7022, #26900 ) ;
#23842=VECTOR ( 'NONE', #36284, 1000.000000000000000 ) ;
#23879=ORIENTED_EDGE ( 'NONE', *, *, #11143, .F. ) ;
#23882=CARTESIAN_POINT ( 'NONE',  ( 34.00000000000000000, -103.4105893997321743, 32.50000000000000000 ) ) ;
#23906=DIRECTION ( 'NONE',  ( -0.000000000000000000, -0.000000000000000000, -1.000000000000000000 ) ) ;
#23936=CARTESIAN_POINT ( 'NONE',  ( -2.308176576174226117E-14, -5.999999999999947597, 27.50000000000000000 ) ) ;
#23946=CARTESIAN_POINT ( 'NONE',  ( 40.99999999999999289, -103.4105893997321743, 32.50000000000000000 ) ) ;
#23948=LINE ( 'NONE', #34821, #29627 ) ;
#23965=VECTOR ( 'NONE', #22586, 1000.000000000000000 ) ;
#23970=AXIS2_PLACEMENT_3D ( 'NONE', #17994, #18165, #3916 ) ;
#23979=ORIENTED_EDGE ( 'NONE', *, *, #14504, .F. ) ;
#23988=FACE_OUTER_BOUND ( 'NONE', #1297, .T. ) ;
#23993=ORIENTED_EDGE ( 'NONE', *, *, #29026, .F. ) ;
#24000=CARTESIAN_POINT ( 'NONE',  ( -4.242640687119211051, 4.242640687119288323, 27.50000000000000000 ) ) ;
#24011=CARTESIAN_POINT ( 'NONE',  ( -108.3061974404896262, 19.22934205795090534, 32.50000000000000000 ) ) ;
#24023=DIRECTION ( 'NONE',  ( 1.000000000000000000, 1.850371707708594366E-15, 0.000000000000000000 ) ) ;
#24025=ORIENTED_EDGE ( 'NONE', *, *, #6303, .T. ) ;
#24047=VERTEX_POINT ( 'NONE', #34876 ) ;
#24048=APPLICATION_CONTEXT ( 'automotive_design' ) ;
#24076=DIRECTION ( 'NONE',  ( -0.000000000000000000, -0.000000000000000000, -1.000000000000000000 ) ) ;
#24079=ORIENTED_EDGE ( 'NONE', *, *, #24532, .T. ) ;
#24080=DIRECTION ( 'NONE',  ( 1.000000000000000000, 0.000000000000000000, 0.000000000000000000 ) ) ;
#24105=EDGE_CURVE ( 'NONE', #36485, #32044, #19666, .T. ) ;
#24120=ORIENTED_EDGE ( 'NONE', *, *, #27181, .T. ) ;
#24127=DIRECTION ( 'NONE',  ( 0.000000000000000000, 0.000000000000000000, 1.000000000000000000 ) ) ;
#24140=CARTESIAN_POINT ( 'NONE',  ( -97.64030476177397588, 67.22390783198484598, 32.50000000000000000 ) ) ;
#24152=ORIENTED_EDGE ( 'NONE', *, *, #26869, .F. ) ;
#24164=ORIENTED_EDGE ( 'NONE', *, *, #25901, .T. ) ;
#24166=ORIENTED_EDGE ( 'NONE', *, *, #24988, .F. ) ;
#24180=CARTESIAN_POINT ( 'NONE',  ( 101.8360233522598719, -31.92205067127980200, 32.50000000000001421 ) ) ;
#24186=CARTESIAN_POINT ( 'NONE',  ( 111.8061974404897825, -19.22934205795014151, 27.50000000000000000 ) ) ;
#24192=DIRECTION ( 'NONE',  ( -0.000000000000000000, -0.000000000000000000, 1.000000000000000000 ) ) ;
#24234=ORIENTED_EDGE ( 'NONE', *, *, #35783, .F. ) ;
#24237=DIRECTION ( 'NONE',  ( -0.000000000000000000, -0.000000000000000000, 1.000000000000000000 ) ) ;
#24257=DIRECTION ( 'NONE',  ( 1.000000000000000000, 0.000000000000000000, 0.000000000000000000 ) ) ;
#24258=CARTESIAN_POINT ( 'NONE',  ( 0.000000000000000000, 0.000000000000000000, 27.50000000000000000 ) ) ;
#24267=VECTOR ( 'NONE', #31771, 1000.000000000000000 ) ;
#24290=DIRECTION ( 'NONE',  ( 1.000000000000000000, 0.000000000000000000, 0.000000000000000000 ) ) ;
#24305=DIRECTION ( 'NONE',  ( -0.000000000000000000, -0.000000000000000000, 1.000000000000000000 ) ) ;
#24309=DIRECTION ( 'NONE',  ( -0.000000000000000000, -0.000000000000000000, -1.000000000000000000 ) ) ;
#24317=DIRECTION ( 'NONE',  ( 1.000000000000000000, -1.850371707708594366E-15, 0.000000000000000000 ) ) ;
#24331=CARTESIAN_POINT ( 'NONE',  ( -82.47399748121956975, 72.51968985770598408, 32.50000000000001421 ) ) ;
#24332=AXIS2_PLACEMENT_3D ( 'NONE', #11754, #20955, #20393 ) ;
#24334=AXIS2_PLACEMENT_3D ( 'NONE', #5141, #25036, #16580 ) ;
#24341=ORIENTED_EDGE ( 'NONE', *, *, #34953, .T. ) ;
#24352=DIRECTION ( 'NONE',  ( 1.000000000000000000, 0.000000000000000000, 0.000000000000000000 ) ) ;
#24354=ORIENTED_EDGE ( 'NONE', *, *, #7907, .T. ) ;
#24378=CYLINDRICAL_SURFACE ( 'NONE', #16600, 3.500000000000003109 ) ;
#24385=AXIS2_PLACEMENT_3D ( 'NONE', #17717, #15095, #31941 ) ;
#24388=CARTESIAN_POINT ( 'NONE',  ( -67.30619744048885877, 84.18124734178336155, 27.50000000000000000 ) ) ;
#24413=CARTESIAN_POINT ( 'NONE',  ( 4.242640687119292764, 4.242640687119187071, 32.50000000000000000 ) ) ;
#24433=FACE_OUTER_BOUND ( 'NONE', #1458, .T. ) ;
#24445=DIRECTION ( 'NONE',  ( -0.7071067811865539010, -0.7071067811865411334, 0.000000000000000000 ) ) ;
#24447=EDGE_CURVE ( 'NONE', #37014, #27017, #16702, .T. ) ;
#24453=EDGE_CURVE ( 'NONE', #3457, #30601, #23516, .T. ) ;
#24457=LINE ( 'NONE', #26694, #17464 ) ;
#24467=DIRECTION ( 'NONE',  ( 1.000000000000000000, 9.251858538542971828E-16, 0.000000000000000000 ) ) ;
#24474=CARTESIAN_POINT ( 'NONE',  ( 110.2237710830536770, 101.7384897088147397, 27.50000000000000000 ) ) ;
#24482=ORIENTED_EDGE ( 'NONE', *, *, #6661, .T. ) ;
#24486=ORIENTED_EDGE ( 'NONE', *, *, #21822, .T. ) ;
#24503=DIRECTION ( 'NONE',  ( 1.000000000000000000, 0.000000000000000000, 0.000000000000000000 ) ) ;
#24521=CARTESIAN_POINT ( 'NONE',  ( 101.4249800177814933, 31.43204461043894327, 27.50000000000000000 ) ) ;
#24532=EDGE_CURVE ( 'NONE', #5973, #2865, #5334, .T. ) ;
#24551=DIRECTION ( 'NONE',  ( -0.000000000000000000, 0.000000000000000000, -1.000000000000000000 ) ) ;
#24561=VERTEX_POINT ( 'NONE', #15077 ) ;
#24562=EDGE_LOOP ( 'NONE', ( #248, #29757, #29403, #24695 ) ) ;
#24583=VERTEX_POINT ( 'NONE', #23346 ) ;
#24628=VERTEX_POINT ( 'NONE', #7206 ) ;
#24665=FACE_OUTER_BOUND ( 'NONE', #8748, .T. ) ;
#24692=DIRECTION ( 'NONE',  ( 0.000000000000000000, 0.000000000000000000, 1.000000000000000000 ) ) ;
#24695=ORIENTED_EDGE ( 'NONE', *, *, #20366, .T. ) ;
#24698=DIRECTION ( 'NONE',  ( -0.000000000000000000, -0.000000000000000000, -1.000000000000000000 ) ) ;
#24706=CARTESIAN_POINT ( 'NONE',  ( -95.78743416778654307, 68.56885790715003282, 32.50000000000000000 ) ) ;
#24723=EDGE_CURVE ( 'NONE', #20815, #7230, #33517, .T. ) ;
#24752=FACE_OUTER_BOUND ( 'NONE', #2397, .T. ) ;
#24777=DIRECTION ( 'NONE',  ( -0.000000000000000000, -0.000000000000000000, -1.000000000000000000 ) ) ;
#24782=ADVANCED_FACE ( 'NONE', ( #25365 ), #27621, .F. ) ;
#24800=EDGE_CURVE ( 'NONE', #17212, #4310, #16561, .T. ) ;
#24802=ORIENTED_EDGE ( 'NONE', *, *, #29357, .T. ) ;
#24813=B_SPLINE_CURVE_WITH_KNOTS ( 'NONE', 3,
 ( #33327, #7838, #27126, #19093, #21522, #30522, #4840, #19267, #36139, #4276, #16269, #1831, #24889, #12870, #36331, #24140, #9886, #24706, #32765, #35972, #4451, #27686, #24331, #10641, #32959, #4649, #7271, #12685 ),
 .UNSPECIFIED., .F., .F.,
 ( 4, 2, 2, 1, 1, 2, 2, 1, 2, 2, 1, 1, 2, 2, 1, 2, 4 ),
 ( 0.1667295141962928384, 0.1840819284725213056, 0.1927581356106355948, 0.2014343427487499116, 0.2361391713012070959, 0.2448153784393213295, 0.2534915855774355076, 0.2708439998536639748, 0.3055488284061209647, 0.3142250355442351983, 0.3229012426823494319, 0.3402536569585778992, 0.3749584855110348336, 0.4096633140634917125, 0.4270157283397201242, 0.4356919354778343578, 0.4443681426159485914 ),
 .UNSPECIFIED. ) ;
#24817=DIRECTION ( 'NONE',  ( -1.000000000000000000, 0.000000000000000000, 0.000000000000000000 ) ) ;
#24821=AXIS2_PLACEMENT_3D ( 'NONE', #22990, #8734, #12078 ) ;
#24834=EDGE_LOOP ( 'NONE', ( #34816, #677, #28246, #9531 ) ) ;
#24846=ORIENTED_EDGE ( 'NONE', *, *, #15362, .T. ) ;
#24852=EDGE_LOOP ( 'NONE', ( #27852, #32013 ) ) ;
#24871=CARTESIAN_POINT ( 'NONE',  ( 82.27241335952179213, 47.49999999999982236, 32.50002500000000083 ) ) ;
#24888=DIRECTION ( 'NONE',  ( -0.000000000000000000, -0.000000000000000000, -1.000000000000000000 ) ) ;
#24889=CARTESIAN_POINT ( 'NONE',  ( -101.6272589138252442, 63.51387141301889727, 32.49999999999999289 ) ) ;
#24918=AXIS2_PLACEMENT_3D ( 'NONE', #4388, #9817, #24080 ) ;
#24921=VERTEX_POINT ( 'NONE', #6348 ) ;
#24936=CARTESIAN_POINT ( 'NONE',  ( -37.50000000000000000, -103.4105893997321743, 32.50000000000000000 ) ) ;
#24940=ORIENTED_EDGE ( 'NONE', *, *, #3763, .F. ) ;
#24966=ORIENTED_EDGE ( 'NONE', *, *, #23758, .T. ) ;
#24975=CARTESIAN_POINT ( 'NONE',  ( -145.0000000000000568, 1.518182058997189877E-12, 27.50000000000000000 ) ) ;
#24988=EDGE_CURVE ( 'NONE', #27017, #10608, #31692, .T. ) ;
#25010=VERTEX_POINT ( 'NONE', #18556 ) ;
#25012=CARTESIAN_POINT ( 'NONE',  ( -70.80619744049063513, -84.18124734178186941, 27.50000000000000000 ) ) ;
#25015=AXIS2_PLACEMENT_3D ( 'NONE', #34232, #33846, #19602 ) ;
#25016=VECTOR ( 'NONE', #8970, 1000.000000000000000 ) ;
#25018=ADVANCED_FACE ( 'NONE', ( #35802 ), #16289, .F. ) ;
#25030=CARTESIAN_POINT ( 'NONE',  ( 23.49188653442568864, 103.5527583403323035, 27.49999400000000094 ) ) ;
#25036=DIRECTION ( 'NONE',  ( -0.000000000000000000, -0.000000000000000000, 1.000000000000000000 ) ) ;
#25043=AXIS2_PLACEMENT_3D ( 'NONE', #6062, #17487, #36644 ) ;
#25051=CARTESIAN_POINT ( 'NONE',  ( 106.7731239591688848, 98.28784258492994752, 32.55002500000000509 ) ) ;
#25067=DIRECTION ( 'NONE',  ( -0.000000000000000000, -0.000000000000000000, -1.000000000000000000 ) ) ;
#25080=ORIENTED_EDGE ( 'NONE', *, *, #12876, .T. ) ;
#25084=LINE ( 'NONE', #30854, #30273 ) ;
#25097=CARTESIAN_POINT ( 'NONE',  ( -34.00000000000000000, 103.4105893997321743, 32.50000000000000000 ) ) ;
#25117=CARTESIAN_POINT ( 'NONE',  ( -55.27226924886021919, 77.26562141134635908, 27.50000000000000000 ) ) ;
#25120=ORIENTED_EDGE ( 'NONE', *, *, #24723, .F. ) ;
#25131=CARTESIAN_POINT ( 'NONE',  ( 88.03900239164613595, -71.83446256730503876, 32.49999999999999289 ) ) ;
#25151=ORIENTED_EDGE ( 'NONE', *, *, #4957, .F. ) ;
#25157=CIRCLE ( 'NONE', #11379, 150.0000000000000284 ) ;
#25176=DIRECTION ( 'NONE',  ( 1.000000000000000000, -3.846960960290410782E-15, 0.000000000000000000 ) ) ;
#25184=DIRECTION ( 'NONE',  ( 0.000000000000000000, 0.000000000000000000, 1.000000000000000000 ) ) ;
#25196=ORIENTED_EDGE ( 'NONE', *, *, #7587, .F. ) ;
#25198=CARTESIAN_POINT ( 'NONE',  ( 5.999999999999998224, 145.0000000000000568, 32.50000000000000000 ) ) ;
#25225=CYLINDRICAL_SURFACE ( 'NONE', #16380, 6.000000000000005329 ) ;
#25243=CARTESIAN_POINT ( 'NONE',  ( 72.72667006429115588, 101.6652913307178636, 32.50000000000000000 ) ) ;
#25246=DIRECTION ( 'NONE',  ( -0.000000000000000000, -0.000000000000000000, -1.000000000000000000 ) ) ;
#25252=ORIENTED_EDGE ( 'NONE', *, *, #21716, .T. ) ;
#25255=FACE_OUTER_BOUND ( 'NONE', #22264, .T. ) ;
#25268=VECTOR ( 'NONE', #33449, 1000.000000000000000 ) ;
#25270=EDGE_LOOP ( 'NONE', ( #12356, #13747, #22751, #17969 ) ) ;
#25274=VECTOR ( 'NONE', #14461, 1000.000000000000000 ) ;
#25276=DIRECTION ( 'NONE',  ( -0.000000000000000000, -0.000000000000000000, -1.000000000000000000 ) ) ;
#25296=CARTESIAN_POINT ( 'NONE',  ( 97.20652429509418369, -67.55932235215701098, 32.50000000000000711 ) ) ;
#25297=CARTESIAN_POINT ( 'NONE',  ( 77.93337651276290501, -72.12094976675109592, 32.50001250000000397 ) ) ;
#25305=CARTESIAN_POINT ( 'NONE',  ( 102.5304832720488832, -102.5304832720499633, 32.55002500000000509 ) ) ;
#25334=CARTESIAN_POINT ( 'NONE',  ( -72.72667006428976322, 101.6652913307188868, 32.50000000000000000 ) ) ;
#25348=CARTESIAN_POINT ( 'NONE',  ( -107.0890852396554891, -43.89229305394454173, 32.50000000000001421 ) ) ;
#25349=ORIENTED_EDGE ( 'NONE', *, *, #6260, .F. ) ;
#25351=VECTOR ( 'NONE', #15432, 1000.000000000000000 ) ;
#25353=AXIS2_PLACEMENT_3D ( 'NONE', #25305, #8047, #11234 ) ;
#25365=FACE_OUTER_BOUND ( 'NONE', #23234, .T. ) ;
#25398=CARTESIAN_POINT ( 'NONE',  ( 16.35123109063852098, -113.9563289638309413, 32.50000000000000711 ) ) ;
#25451=STYLED_ITEM ( 'NONE', ( #16487 ), #32134 ) ;
#25473=CARTESIAN_POINT ( 'NONE',  ( 86.78973740846132046, -72.09873635328332853, 32.50000000000000000 ) ) ;
#25474=CARTESIAN_POINT ( 'NONE',  ( -103.8785218410652647, -60.08491969753902850, 32.50000000000000000 ) ) ;
#25478=DIRECTION ( 'NONE',  ( 0.000000000000000000, 0.000000000000000000, 1.000000000000000000 ) ) ;
#25494=ORIENTED_EDGE ( 'NONE', *, *, #30481, .T. ) ;
#25503=AXIS2_PLACEMENT_3D ( 'NONE', #20222, #11761, #23578 ) ;
#25522=ORIENTED_EDGE ( 'NONE', *, *, #32675, .T. ) ;
#25525=VERTEX_POINT ( 'NONE', #7067 ) ;
#25529=VECTOR ( 'NONE', #33600, 1000.000000000000000 ) ;
#25530=CARTESIAN_POINT ( 'NONE',  ( 37.50000000000000000, -103.4105893997321743, 27.50000000000000000 ) ) ;
#25533=( GEOMETRIC_REPRESENTATION_CONTEXT ( 3 ) GLOBAL_UNCERTAINTY_ASSIGNED_CONTEXT ( ( #8053 ) ) GLOBAL_UNIT_ASSIGNED_CONTEXT ( ( #16328, #7330, #3168 ) ) REPRESENTATION_CONTEXT ( 'NONE', 'WORKASPACE' ) );
#25538=EDGE_CURVE ( 'NONE', #18383, #12647, #34743, .T. ) ;
#25545=DIRECTION ( 'NONE',  ( 1.000000000000000000, 0.000000000000000000, 0.000000000000000000 ) ) ;
#25554=AXIS2_PLACEMENT_3D ( 'NONE', #2119, #16376, #13755 ) ;
#25559=CYLINDRICAL_SURFACE ( 'NONE', #25554, 95.00000000000001421 ) ;
#25570=CARTESIAN_POINT ( 'NONE',  ( -2.545082869045428353, 120.0000000191570990, 27.49998800000000188 ) ) ;
#25572=ORIENTED_EDGE ( 'NONE', *, *, #28591, .T. ) ;
#25573=CYLINDRICAL_SURFACE ( 'NONE', #25043, 30.00000000000000000 ) ;
#25574=DIRECTION ( 'NONE',  ( -0.000000000000000000, -0.000000000000000000, 1.000000000000000000 ) ) ;
#25605=PLANE ( 'NONE',  #26670 ) ;
#25608=LINE ( 'NONE', #10800, #16494 ) ;
#25626=FACE_OUTER_BOUND ( 'NONE', #21245, .T. ) ;
#25631=VERTEX_POINT ( 'NONE', #28394 ) ;
#25637=EDGE_LOOP ( 'NONE', ( #2822, #23601 ) ) ;
#25644=CARTESIAN_POINT ( 'NONE',  ( 0.000000000000000000, 0.000000000000000000, 27.50000000000000000 ) ) ;
#25653=CARTESIAN_POINT ( 'NONE',  ( 102.5304832720496080, 102.5304832720492527, 32.55002500000000509 ) ) ;
#25672=EDGE_CURVE ( 'NONE', #24561, #33879, #20719, .T. ) ;
#25677=CARTESIAN_POINT ( 'NONE',  ( 107.1783900501392139, -49.76387890855416885, 32.50000000000000711 ) ) ;
#25678=CARTESIAN_POINT ( 'NONE',  ( -82.47367650156751040, -72.51972198845571427, 32.50000000000000711 ) ) ;
#25739=AXIS2_PLACEMENT_3D ( 'NONE', #27281, #2155, #24290 ) ;
#25743=PLANE ( 'NONE',  #32737 ) ;
#25777=VERTEX_POINT ( 'NONE', #26513 ) ;
#25778=CARTESIAN_POINT ( 'NONE',  ( -124.4080600076929954, 12.15049814296761888, 27.50000000000000000 ) ) ;
#25786=LINE ( 'NONE', #25051, #31126 ) ;
#25795=CARTESIAN_POINT ( 'NONE',  ( -94.55012560584690107, -9.234378588653415321, 27.50000000000000000 ) ) ;
#25812=DIRECTION ( 'NONE',  ( 0.000000000000000000, 0.000000000000000000, 1.000000000000000000 ) ) ;
#25833=CARTESIAN_POINT ( 'NONE',  ( 0.000000000000000000, 0.000000000000000000, 27.50000000000000000 ) ) ;
#25835=DIRECTION ( 'NONE',  ( -1.000000000000000000, 0.000000000000000000, 0.000000000000000000 ) ) ;
#25839=LINE ( 'NONE', #25117, #28626 ) ;
#25847=CYLINDRICAL_SURFACE ( 'NONE', #15772, 95.00000000000001421 ) ;
#25848=CARTESIAN_POINT ( 'NONE',  ( 107.3056136255987809, -47.85537046088835211, 32.50000000000000000 ) ) ;
#25849=DIRECTION ( 'NONE',  ( 0.000000000000000000, 0.000000000000000000, 1.000000000000000000 ) ) ;
#25858=CARTESIAN_POINT ( 'NONE',  ( 149.8799519615616020, -6.000000000000508038, 32.50000000000000000 ) ) ;
#25860=EDGE_CURVE ( 'NONE', #7230, #13311, #36259, .T. ) ;
#25868=CARTESIAN_POINT ( 'NONE',  ( 6.000000000000000000, -145.0000000000000568, 32.55002500000000509 ) ) ;
#25882=LINE ( 'NONE', #8820, #8416 ) ;
#25899=FACE_BOUND ( 'NONE', #6872, .T. ) ;
#25901=EDGE_CURVE ( 'NONE', #16892, #31169, #16533, .T. ) ;
#25916=CARTESIAN_POINT ( 'NONE',  ( 0.000000000000000000, 0.000000000000000000, 27.50000000000000000 ) ) ;
#25930=EDGE_CURVE ( 'NONE', #16096, #7521, #17181, .T. ) ;
#25933=ORIENTED_EDGE ( 'NONE', *, *, #34210, .F. ) ;
#25938=DIRECTION ( 'NONE',  ( -0.000000000000000000, -0.000000000000000000, 1.000000000000000000 ) ) ;
#25945=FACE_OUTER_BOUND ( 'NONE', #22587, .T. ) ;
#25950=CARTESIAN_POINT ( 'NONE',  ( -23.27275137504124203, -104.1535408905101860, 32.50000000000000711 ) ) ;
#25951=ORIENTED_EDGE ( 'NONE', *, *, #24532, .F. ) ;
#25971=DIRECTION ( 'NONE',  ( 0.000000000000000000, 0.000000000000000000, 1.000000000000000000 ) ) ;
#25987=VECTOR ( 'NONE', #7268, 1000.000000000000000 ) ;
#26024=CIRCLE ( 'NONE', #3888, 3.500000000000003109 ) ;
#26030=ADVANCED_FACE ( 'NONE', ( #22556 ), #25559, .F. ) ;
#26071=ORIENTED_EDGE ( 'NONE', *, *, #18406, .T. ) ;
#26078=DIRECTION ( 'NONE',  ( -0.000000000000000000, -0.000000000000000000, 1.000000000000000000 ) ) ;
#26121=ORIENTED_EDGE ( 'NONE', *, *, #35783, .T. ) ;
#26138=CARTESIAN_POINT ( 'NONE',  ( 70.80619744049005249, 84.18124734178236679, 32.50000000000000000 ) ) ;
#26144=DIRECTION ( 'NONE',  ( 0.000000000000000000, 0.000000000000000000, 1.000000000000000000 ) ) ;
#26146=AXIS2_PLACEMENT_3D ( 'NONE', #2735, #25812, #11530 ) ;
#26149=CARTESIAN_POINT ( 'NONE',  ( -101.7384897088158766, -110.2237710830526112, 32.55002500000000509 ) ) ;
#26157=CARTESIAN_POINT ( 'NONE',  ( -72.72667006428976322, 101.6652913307188868, 27.50000000000000000 ) ) ;
#26174=CARTESIAN_POINT ( 'NONE',  ( 106.7731239591682026, -98.28784258493070070, 32.55002500000000509 ) ) ;
#26186=AXIS2_PLACEMENT_3D ( 'NONE', #35843, #12573, #35295 ) ;
#26196=LINE ( 'NONE', #28980, #31444 ) ;
#26200=ORIENTED_EDGE ( 'NONE', *, *, #20100, .T. ) ;
#26204=VECTOR ( 'NONE', #20398, 1000.000000000000000 ) ;
#26205=ORIENTED_EDGE ( 'NONE', *, *, #26843, .F. ) ;
#26206=AXIS2_PLACEMENT_3D ( 'NONE', #19912, #11096, #14094 ) ;
#26225=CARTESIAN_POINT ( 'NONE',  ( 0.000000000000000000, 0.000000000000000000, 27.50000000000000000 ) ) ;
#26246=CARTESIAN_POINT ( 'NONE',  ( -37.50000000000000000, -103.4105893997321743, 32.50000000000000000 ) ) ;
#26250=CARTESIAN_POINT ( 'NONE',  ( 106.4067350097334099, 40.94759250334365674, 32.50000000000000000 ) ) ;
#26260=DIRECTION ( 'NONE',  ( -0.000000000000000000, -0.000000000000000000, -1.000000000000000000 ) ) ;
#26278=CIRCLE ( 'NONE', #31072, 25.00000000000000000 ) ;
#26282=CIRCLE ( 'NONE', #19703, 6.000000000000005329 ) ;
#26286=LINE ( 'NONE', #12011, #28618 ) ;
#26296=EDGE_CURVE ( 'NONE', #27651, #23728, #10625, .T. ) ;
#26298=AXIS2_PLACEMENT_3D ( 'NONE', #22276, #33349, #24352 ) ;
#26311=AXIS2_PLACEMENT_3D ( 'NONE', #25644, #14550, #16834 ) ;
#26316=ADVANCED_FACE ( 'NONE', ( #35854 ), #18605, .F. ) ;
#26341=VECTOR ( 'NONE', #9753, 1000.000000000000000 ) ;
#26345=EDGE_CURVE ( 'NONE', #15626, #17730, #27022, .T. ) ;
#26348=CYLINDRICAL_SURFACE ( 'NONE', #16095, 25.00000000000000711 ) ;
#26358=ORIENTED_EDGE ( 'NONE', *, *, #19700, .F. ) ;
#26371=ORIENTED_EDGE ( 'NONE', *, *, #1567, .F. ) ;
#26384=DIRECTION ( 'NONE',  ( 0.000000000000000000, -0.000000000000000000, -1.000000000000000000 ) ) ;
#26387=EDGE_CURVE ( 'NONE', #9129, #35778, #15411, .T. ) ;
#26394=ORIENTED_EDGE ( 'NONE', *, *, #3901, .T. ) ;
#26405=EDGE_LOOP ( 'NONE', ( #5985, #21231, #29906, #7705 ) ) ;
#26430=CARTESIAN_POINT ( 'NONE',  ( 106.3598707460134989, 54.82082426949677512, 32.50000000000000000 ) ) ;
#26445=CARTESIAN_POINT ( 'NONE',  ( -101.4249800177817207, -31.43204461043823272, 32.50002500000000083 ) ) ;
#26452=ORIENTED_EDGE ( 'NONE', *, *, #32497, .F. ) ;
#26461=CARTESIAN_POINT ( 'NONE',  ( -106.0139304841753329, 39.63070125058630566, 32.50000000000000000 ) ) ;
#26482=ORIENTED_EDGE ( 'NONE', *, *, #13643, .T. ) ;
#26489=DIRECTION ( 'NONE',  ( -1.000000000000000000, 0.000000000000000000, 0.000000000000000000 ) ) ;
#26493=CARTESIAN_POINT ( 'NONE',  ( 10.49241169935725537, -117.7011479744511746, 32.50000000000000000 ) ) ;
#26495=CARTESIAN_POINT ( 'NONE',  ( -94.55012560584668790, 9.234378588655390629, 27.50000000000000000 ) ) ;
#26497=EDGE_CURVE ( 'NONE', #31244, #16882, #27754, .T. ) ;
#26505=ADVANCED_FACE ( 'NONE', ( #16887 ), #13324, .F. ) ;
#26513=CARTESIAN_POINT ( 'NONE',  ( -55.27226924886021919, 77.26562141134635908, 32.50000000000000000 ) ) ;
#26524=DIRECTION ( 'NONE',  ( 0.000000000000000000, 0.000000000000000000, 1.000000000000000000 ) ) ;
#26526=DIRECTION ( 'NONE',  ( 1.000000000000000000, 0.000000000000000000, 0.000000000000000000 ) ) ;
#26557=LINE ( 'NONE', #12855, #3480 ) ;
#26578=CYLINDRICAL_SURFACE ( 'NONE', #9787, 30.00000000000000000 ) ;
#26582=ORIENTED_EDGE ( 'NONE', *, *, #30935, .T. ) ;
#26597=EDGE_CURVE ( 'NONE', #10948, #28579, #1456, .T. ) ;
#26603=AXIS2_PLACEMENT_3D ( 'NONE', #15009, #9741, #17612 ) ;
#26605=ORIENTED_EDGE ( 'NONE', *, *, #11258, .T. ) ;
#26608=DIRECTION ( 'NONE',  ( 0.000000000000000000, 0.000000000000000000, 1.000000000000000000 ) ) ;
#26629=FACE_BOUND ( 'NONE', #6168, .T. ) ;
#26641=VECTOR ( 'NONE', #26991, 1000.000000000000000 ) ;
#26650=ORIENTED_EDGE ( 'NONE', *, *, #27860, .F. ) ;
#26655=DIRECTION ( 'NONE',  ( 1.000000000000000000, 0.000000000000000000, 0.000000000000000000 ) ) ;
#26660=CARTESIAN_POINT ( 'NONE',  ( 0.000000000000000000, 0.000000000000000000, 27.50000000000000000 ) ) ;
#26661=B_SPLINE_CURVE_WITH_KNOTS ( 'NONE', 3,
 ( #19402, #5526, #30821, #34227, #16597, #8352, #31027, #16792, #13950, #25398, #34042, #19788, #26493, #35340, #11679, #23136, #3255, #805, #6632, #14684, #3637, #11873, #10149, #34589, #15065, #18060, #29481, #440, #8889, #3803, #3454, #14512, #31748, #25950, #23333 ),
 .UNSPECIFIED., .F., .F.,
 ( 4, 2, 1, 1, 2, 2, 1, 2, 2, 2, 2, 1, 2, 2, 1, 2, 2, 1, 1, 2, 4 ),
 ( 0.05563282717588803605, 0.06778080578339820694, 0.07992878439090839171, 0.1042247416059285114, 0.1163727202134385852, 0.1285206988209486867, 0.1528166560359688342, 0.1771126132509889817, 0.1892605918584991387, 0.2014085704660092402, 0.2500004848960496462, 0.2985923993260899412, 0.3107403779336000427, 0.3228883565411101442, 0.3471843137561303472, 0.3714802709711505502, 0.3836282495786607072, 0.3957762281861708642, 0.4200721854011910117, 0.4322201640087010577, 0.4443681426162111037 ),
 .UNSPECIFIED. ) ;
#26664=LINE ( 'NONE', #17666, #11832 ) ;
#26670=AXIS2_PLACEMENT_3D ( 'NONE', #30830, #2715, #16414 ) ;
#26677=CIRCLE ( 'NONE', #29662, 95.00000000000001421 ) ;
#26694=CARTESIAN_POINT ( 'NONE',  ( 5.999999999999985789, 149.8799519615616305, 32.55002500000000509 ) ) ;
#26695=CARTESIAN_POINT ( 'NONE',  ( -23.49154088336464241, 103.5526315789473699, 32.50000000000000000 ) ) ;
#26705=AXIS2_PLACEMENT_3D ( 'NONE', #6675, #35190, #10046 ) ;
#26730=CARTESIAN_POINT ( 'NONE',  ( -4.242640687119340726, -4.242640687119236809, 27.50000000000000000 ) ) ;
#26745=VECTOR ( 'NONE', #15067, 1000.000000000000000 ) ;
#26755=VERTEX_POINT ( 'NONE', #10812 ) ;
#26761=DIRECTION ( 'NONE',  ( 0.000000000000000000, 0.000000000000000000, 1.000000000000000000 ) ) ;
#26763=EDGE_CURVE ( 'NONE', #27222, #4461, #17615, .T. ) ;
#26765=DIRECTION ( 'NONE',  ( 0.000000000000000000, 0.000000000000000000, 1.000000000000000000 ) ) ;
#26787=AXIS2_PLACEMENT_3D ( 'NONE', #11955, #29201, #31815 ) ;
#26794=ORIENTED_EDGE ( 'NONE', *, *, #812, .T. ) ;
#26797=EDGE_CURVE ( 'NONE', #15626, #9129, #1673, .T. ) ;
#26798=ORIENTED_EDGE ( 'NONE', *, *, #29393, .F. ) ;
#26802=EDGE_CURVE ( 'NONE', #32886, #24047, #27197, .T. ) ;
#26825=CARTESIAN_POINT ( 'NONE',  ( 67.30619744048945563, -84.18124734178287838, 32.50000000000000000 ) ) ;
#26835=CYLINDRICAL_SURFACE ( 'NONE', #26186, 150.0000000000000284 ) ;
#26843=EDGE_CURVE ( 'NONE', #16830, #11964, #19429, .T. ) ;
#26869=EDGE_CURVE ( 'NONE', #22692, #8483, #5663, .T. ) ;
#26870=EDGE_LOOP ( 'NONE', ( #16535, #8697, #26200, #1238, #29659, #5670, #23699, #19778, #25196, #22812, #28167, #18456, #15068, #34489, #3138, #28083, #2782, #14881, #13287, #16498, #5510, #9633, #16163, #12988, #20081, #24354, #16763, #9636, #25572 ) ) ;
#26874=LINE ( 'NONE', #3630, #25351 ) ;
#26876=ORIENTED_EDGE ( 'NONE', *, *, #33907, .F. ) ;
#26900=DIRECTION ( 'NONE',  ( 1.000000000000000000, 0.000000000000000000, 0.000000000000000000 ) ) ;
#26901=DIRECTION ( 'NONE',  ( 0.000000000000000000, 0.000000000000000000, 1.000000000000000000 ) ) ;
#26910=CARTESIAN_POINT ( 'NONE',  ( -5.999999999999947597, 2.132877728683645235E-15, 27.50000000000000000 ) ) ;
#26915=AXIS2_PLACEMENT_3D ( 'NONE', #21302, #24305, #6511 ) ;
#26918=CARTESIAN_POINT ( 'NONE',  ( 0.000000000000000000, 0.000000000000000000, 27.50000000000000000 ) ) ;
#26927=DIRECTION ( 'NONE',  ( -0.000000000000000000, -0.000000000000000000, 1.000000000000000000 ) ) ;
#26931=CARTESIAN_POINT ( 'NONE',  ( 98.28784258492957804, -106.7731239591692116, 32.55002500000000509 ) ) ;
#26932=AXIS2_PLACEMENT_3D ( 'NONE', #1381, #12803, #24257 ) ;
#26953=EDGE_CURVE ( 'NONE', #12647, #23824, #30225, .T. ) ;
#26955=DIRECTION ( 'NONE',  ( -3.554796214472773777E-16, -1.000000000000000000, 0.000000000000000000 ) ) ;
#26977=CIRCLE ( 'NONE', #17403, 95.00000000000001421 ) ;
#26982=EDGE_CURVE ( 'NONE', #1442, #30601, #32633, .T. ) ;
#26984=CARTESIAN_POINT ( 'NONE',  ( -98.28784258492883907, 106.7731239591698937, 32.55002500000000509 ) ) ;
#26990=ORIENTED_EDGE ( 'NONE', *, *, #16806, .F. ) ;
#26991=DIRECTION ( 'NONE',  ( -0.000000000000000000, -0.000000000000000000, 1.000000000000000000 ) ) ;
#26993=DIRECTION ( 'NONE',  ( -0.000000000000000000, -0.000000000000000000, -1.000000000000000000 ) ) ;
#27017=VERTEX_POINT ( 'NONE', #37057 ) ;
#27022=LINE ( 'NONE', #24413, #30951 ) ;
#27038=DIRECTION ( 'NONE',  ( 0.000000000000000000, 0.000000000000000000, 1.000000000000000000 ) ) ;
#27039=CARTESIAN_POINT ( 'NONE',  ( -94.55012560584690107, -9.234378588653417097, 27.50000000000000000 ) ) ;
#27050=EDGE_CURVE ( 'NONE', #33855, #4682, #20509, .T. ) ;
#27076=CARTESIAN_POINT ( 'NONE',  ( -34.00000000000000000, -103.4105893997321743, 27.50000000000000000 ) ) ;
#27087=CYLINDRICAL_SURFACE ( 'NONE', #29720, 6.000000000000005329 ) ;
#27094=EDGE_LOOP ( 'NONE', ( #15059, #16070, #33766, #23268 ) ) ;
#27095=FACE_BOUND ( 'NONE', #4687, .T. ) ;
#27123=CARTESIAN_POINT ( 'NONE',  ( -5.999999999999998224, -145.0000000000000568, 32.55002500000000509 ) ) ;
#27126=CARTESIAN_POINT ( 'NONE',  ( -107.2242716242193836, 49.31285668773285380, 32.49999999999999289 ) ) ;
#27131=CARTESIAN_POINT ( 'NONE',  ( 4.242640687119310527, 4.242640687119267007, 27.50000000000000000 ) ) ;
#27139=EDGE_LOOP ( 'NONE', ( #23269, #23532 ) ) ;
#27155=DIRECTION ( 'NONE',  ( 1.000000000000000000, 0.000000000000000000, 0.000000000000000000 ) ) ;
#27168=FACE_OUTER_BOUND ( 'NONE', #15138, .T. ) ;
#27181=EDGE_CURVE ( 'NONE', #6052, #17563, #28431, .T. ) ;
#27182=ORIENTED_EDGE ( 'NONE', *, *, #30847, .F. ) ;
#27184=ORIENTED_EDGE ( 'NONE', *, *, #6583, .T. ) ;
#27197=CIRCLE ( 'NONE', #11640, 30.00000000000000000 ) ;
#27214=VECTOR ( 'NONE', #35430, 1000.000000000000000 ) ;
#27222=VERTEX_POINT ( 'NONE', #27076 ) ;
#27247=DIRECTION ( 'NONE',  ( 1.000000000000000000, 0.000000000000000000, 0.000000000000000000 ) ) ;
#27248=CARTESIAN_POINT ( 'NONE',  ( -101.7384897088135887, 110.2237710830547286, 32.50000000000000000 ) ) ;
#27264=VERTEX_POINT ( 'NONE', #10218 ) ;
#27281=CARTESIAN_POINT ( 'NONE',  ( 0.000000000000000000, 0.000000000000000000, 27.50000000000000000 ) ) ;
#27284=AXIS2_PLACEMENT_3D ( 'NONE', #7905, #2280, #19340 ) ;
#27292=EDGE_CURVE ( 'NONE', #7532, #24583, #29656, .T. ) ;
#27336=CARTESIAN_POINT ( 'NONE',  ( 0.000000000000000000, 0.000000000000000000, 27.50000000000000000 ) ) ;
#27343=VERTEX_POINT ( 'NONE', #17120 ) ;
#27363=CARTESIAN_POINT ( 'NONE',  ( 124.4080600076931375, 12.15049814296589226, 32.50002500000000083 ) ) ;
#27364=DIRECTION ( 'NONE',  ( 1.000000000000000000, 0.000000000000000000, 0.000000000000000000 ) ) ;
#27366=DIRECTION ( 'NONE',  ( 1.000000000000000000, 0.000000000000000000, 0.000000000000000000 ) ) ;
#27370=AXIS2_PLACEMENT_3D ( 'NONE', #29840, #21029, #18776 ) ;
#27371=ORIENTED_EDGE ( 'NONE', *, *, #14217, .F. ) ;
#27396=ORIENTED_EDGE ( 'NONE', *, *, #13092, .T. ) ;
#27416=AXIS2_PLACEMENT_3D ( 'NONE', #3658, #653, #14710 ) ;
#27447=ORIENTED_EDGE ( 'NONE', *, *, #23402, .F. ) ;
#27452=CARTESIAN_POINT ( 'NONE',  ( 51.68138994340220904, -113.8157894736842053, 27.50000000000000000 ) ) ;
#27468=VERTEX_POINT ( 'NONE', #18210 ) ;
#27469=FACE_OUTER_BOUND ( 'NONE', #11937, .T. ) ;
#27474=VECTOR ( 'NONE', #28089, 1000.000000000000000 ) ;
#27478=EDGE_LOOP ( 'NONE', ( #29810, #14469, #11835, #12566 ) ) ;
#27493=ORIENTED_EDGE ( 'NONE', *, *, #29357, .F. ) ;
#27506=CARTESIAN_POINT ( 'NONE',  ( 104.8061974404897683, -19.22934205795014151, 27.50000000000000000 ) ) ;
#27513=DIRECTION ( 'NONE',  ( 0.000000000000000000, 0.000000000000000000, 1.000000000000000000 ) ) ;
#27520=EDGE_CURVE ( 'NONE', #23651, #17786, #17093, .T. ) ;
#27537=DIRECTION ( 'NONE',  ( -0.000000000000000000, -0.000000000000000000, -1.000000000000000000 ) ) ;
#27547=B_SPLINE_CURVE_WITH_KNOTS ( 'NONE', 3,
 ( #16937, #8501, #13932, #19767, #33463, #17121, #2683, #28361, #25570, #33644, #37011, #11318, #5135, #34209, #30630, #19219, #31193, #25030 ),
 .UNSPECIFIED., .F., .F.,
 ( 4, 2, 2, 2, 2, 2, 2, 2, 4 ),
 ( 0.1412743459061075735, 0.2309557491716168476, 0.3206371524371260939, 0.4103185557026353125, 0.4999999589681445311, 0.5896813622336537497, 0.6793627654991629683, 0.7690441687646720759, 0.8587255720301810724 ),
 .UNSPECIFIED. ) ;
#27552=ADVANCED_FACE ( 'NONE', ( #613 ), #12026, .F. ) ;
#27555=VERTEX_POINT ( 'NONE', #32080 ) ;
#27556=EDGE_CURVE ( 'NONE', #12740, #1358, #6418, .T. ) ;
#27586=ORIENTED_EDGE ( 'NONE', *, *, #12272, .T. ) ;
#27606=DIRECTION ( 'NONE',  ( -0.000000000000000000, -0.000000000000000000, 1.000000000000000000 ) ) ;
#27621=CYLINDRICAL_SURFACE ( 'NONE', #37096, 6.000000000000005329 ) ;
#27631=CARTESIAN_POINT ( 'NONE',  ( 77.93343913441695747, 72.12058696850802164, 27.50000000000000000 ) ) ;
#27646=DIRECTION ( 'NONE',  ( -0.000000000000000000, -0.000000000000000000, -1.000000000000000000 ) ) ;
#27651=VERTEX_POINT ( 'NONE', #13162 ) ;
#27652=DIRECTION ( 'NONE',  ( -0.000000000000000000, -0.000000000000000000, -1.000000000000000000 ) ) ;
#27663=DIRECTION ( 'NONE',  ( -0.000000000000000000, -0.000000000000000000, 1.000000000000000000 ) ) ;
#27664=DIRECTION ( 'NONE',  ( 0.000000000000000000, 0.000000000000000000, 1.000000000000000000 ) ) ;
#27667=DIRECTION ( 'NONE',  ( 0.000000000000000000, 0.000000000000000000, 1.000000000000000000 ) ) ;
#27681=AXIS2_PLACEMENT_3D ( 'NONE', #31309, #28146, #2633 ) ;
#27686=CARTESIAN_POINT ( 'NONE',  ( -85.18031014763894859, 72.40127513648181434, 32.50000000000000000 ) ) ;
#27706=DIRECTION ( 'NONE',  ( -0.000000000000000000, -0.000000000000000000, 1.000000000000000000 ) ) ;
#27712=ORIENTED_EDGE ( 'NONE', *, *, #1998, .F. ) ;
#27723=CARTESIAN_POINT ( 'NONE',  ( -79.75043533441352395, -72.37696440020876310, 32.50000000000000000 ) ) ;
#27728=EDGE_LOOP ( 'NONE', ( #9373, #2256, #3893, #17402 ) ) ;
#27729=ORIENTED_EDGE ( 'NONE', *, *, #3313, .T. ) ;
#27730=CARTESIAN_POINT ( 'NONE',  ( -106.7731239591675205, 98.28784258493143966, 32.55002500000000509 ) ) ;
#27754=LINE ( 'NONE', #27949, #8790 ) ;
#27763=DIRECTION ( 'NONE',  ( 1.000000000000000000, 0.000000000000000000, 0.000000000000000000 ) ) ;
#27786=EDGE_CURVE ( 'NONE', #20315, #25777, #33198, .T. ) ;
#27793=VERTEX_POINT ( 'NONE', #5466 ) ;
#27806=DIRECTION ( 'NONE',  ( 1.000000000000000000, 0.000000000000000000, 0.000000000000000000 ) ) ;
#27808=CARTESIAN_POINT ( 'NONE',  ( 0.000000000000000000, 0.000000000000000000, 32.50000000000000000 ) ) ;
#27821=VERTEX_POINT ( 'NONE', #16724 ) ;
#27843=ORIENTED_EDGE ( 'NONE', *, *, #8807, .F. ) ;
#27852=ORIENTED_EDGE ( 'NONE', *, *, #17633, .T. ) ;
#27860=EDGE_CURVE ( 'NONE', #13060, #19610, #36298, .T. ) ;
#27878=AXIS2_PLACEMENT_3D ( 'NONE', #2238, #2794, #8039 ) ;
#27884=ORIENTED_EDGE ( 'NONE', *, *, #6435, .F. ) ;
#27893=DIRECTION ( 'NONE',  ( 1.000000000000000000, 0.000000000000000000, 0.000000000000000000 ) ) ;
#27905=DIRECTION ( 'NONE',  ( -0.000000000000000000, -0.000000000000000000, -1.000000000000000000 ) ) ;
#27910=CARTESIAN_POINT ( 'NONE',  ( -124.4080600076932370, -12.15049814296501829, 27.50000000000000000 ) ) ;
#27930=VERTEX_POINT ( 'NONE', #14616 ) ;
#27949=CARTESIAN_POINT ( 'NONE',  ( 2.094888803305880329E-14, 6.000000000000000000, 32.50000000000000000 ) ) ;
#27963=LINE ( 'NONE', #31318, #34533 ) ;
#27972=CARTESIAN_POINT ( 'NONE',  ( -101.8947384033993018, -31.99217250720169758, 32.50000000000000000 ) ) ;
#27982=DIRECTION ( 'NONE',  ( 0.7071067811865489050, 0.7071067811865461294, -0.000000000000000000 ) ) ;
#27998=EDGE_LOOP ( 'NONE', ( #20579, #17886, #10402, #5829 ) ) ;
#28020=ORIENTED_EDGE ( 'NONE', *, *, #36729, .T. ) ;
#28029=DIRECTION ( 'NONE',  ( 0.000000000000000000, 0.000000000000000000, 1.000000000000000000 ) ) ;
#28043=ORIENTED_EDGE ( 'NONE', *, *, #15148, .F. ) ;
#28083=ORIENTED_EDGE ( 'NONE', *, *, #7149, .T. ) ;
#28089=DIRECTION ( 'NONE',  ( 0.000000000000000000, 0.000000000000000000, 1.000000000000000000 ) ) ;
#28107=AXIS2_PLACEMENT_3D ( 'NONE', #29510, #20704, #29340 ) ;
#28122=ORIENTED_EDGE ( 'NONE', *, *, #12096, .T. ) ;
#28124=EDGE_CURVE ( 'NONE', #36485, #22685, #3925, .T. ) ;
#28146=DIRECTION ( 'NONE',  ( 0.000000000000000000, 0.000000000000000000, 1.000000000000000000 ) ) ;
#28167=ORIENTED_EDGE ( 'NONE', *, *, #8726, .T. ) ;
#28168=CIRCLE ( 'NONE', #11976, 30.00000000000000000 ) ;
#28172=ORIENTED_EDGE ( 'NONE', *, *, #11654, .T. ) ;
#28216=EDGE_CURVE ( 'NONE', #32044, #36485, #26024, .T. ) ;
#28223=CARTESIAN_POINT ( 'NONE',  ( 124.4080600076930665, -12.15049814296675201, 27.50000000000000000 ) ) ;
#28225=DIRECTION ( 'NONE',  ( 0.000000000000000000, 0.000000000000000000, 1.000000000000000000 ) ) ;
#28237=ORIENTED_EDGE ( 'NONE', *, *, #21482, .T. ) ;
#28241=ORIENTED_EDGE ( 'NONE', *, *, #7610, .T. ) ;
#28246=ORIENTED_EDGE ( 'NONE', *, *, #26387, .F. ) ;
#28256=CYLINDRICAL_SURFACE ( 'NONE', #28689, 95.00000000000001421 ) ;
#28257=EDGE_CURVE ( 'NONE', #24628, #16096, #23948, .T. ) ;
#28278=CARTESIAN_POINT ( 'NONE',  ( -98.00106544729364089, -66.93781643011477911, 32.49999999999999289 ) ) ;
#28320=EDGE_CURVE ( 'NONE', #13311, #12717, #32630, .T. ) ;
#28325=FACE_OUTER_BOUND ( 'NONE', #21593, .T. ) ;
#28334=ORIENTED_EDGE ( 'NONE', *, *, #27786, .F. ) ;
#28348=ADVANCED_FACE ( 'NONE', ( #1609 ), #4253, .F. ) ;
#28361=CARTESIAN_POINT ( 'NONE',  ( -5.089798516654387761, 119.6083603441600047, 27.49998800000000543 ) ) ;
#28362=DIRECTION ( 'NONE',  ( -0.000000000000000000, 0.000000000000000000, -1.000000000000000000 ) ) ;
#28369=VERTEX_POINT ( 'NONE', #7614 ) ;
#28394=CARTESIAN_POINT ( 'NONE',  ( 104.8061974404898820, 19.22934205794938478, 27.50000000000000000 ) ) ;
#28398=B_SPLINE_CURVE_WITH_KNOTS ( 'NONE', 3,
 ( #3920, #32422, #35059, #9168, #562, #6178, #9734, #21170, #29037, #17606, #3570, #20600, #17997, #1122, #12346, #23815, #9563, #15175, #3740, #26430, #31842, #32024, #11984, #3374, #32600, #6924, #26250, #34877, #738, #17806, #35268, #12547, #20994, #6735, #29598 ),
 .UNSPECIFIED., .F., .F.,
 ( 4, 2, 1, 1, 2, 2, 1, 2, 2, 2, 2, 1, 2, 2, 1, 2, 2, 1, 1, 2, 4 ),
 ( 0.05563282717590559839, 0.06778080578341673379, 0.07992878439092786225, 0.1042247416059501192, 0.1163727202134613725, 0.1285206988209726398, 0.1528166560359950910, 0.1771126132510175422, 0.1892605918585288927, 0.2014085704660402432, 0.2500004848960857839, 0.2985923993261312415, 0.3107403779336425642, 0.3228883565411538870, 0.3471843137561765325, 0.3714802709711991224, 0.3836282495787105007, 0.3957762281862218789, 0.4200721854012446355, 0.4322201640087560692, 0.4443681426162675030 ),
 .UNSPECIFIED. ) ;
#28399=CYLINDRICAL_SURFACE ( 'NONE', #9430, 25.00000000000000000 ) ;
#28407=CYLINDRICAL_SURFACE ( 'NONE', #26146, 150.0000000000000284 ) ;
#28419=ORIENTED_EDGE ( 'NONE', *, *, #35923, .F. ) ;
#28429=DIRECTION ( 'NONE',  ( 0.000000000000000000, 0.000000000000000000, 1.000000000000000000 ) ) ;
#28431=CIRCLE ( 'NONE', #20635, 150.0000000000000284 ) ;
#28449=FACE_OUTER_BOUND ( 'NONE', #2033, .T. ) ;
#28450=ADVANCED_FACE ( 'NONE', ( #2160 ), #25605, .F. ) ;
#28477=DIRECTION ( 'NONE',  ( 0.000000000000000000, 0.000000000000000000, 1.000000000000000000 ) ) ;
#28479=FILL_AREA_STYLE ('',( #343 ) ) ;
#28494=ORIENTED_EDGE ( 'NONE', *, *, #2709, .F. ) ;
#28499=CARTESIAN_POINT ( 'NONE',  ( 0.000000000000000000, 0.000000000000000000, 32.50000000000000000 ) ) ;
#28544=VERTEX_POINT ( 'NONE', #25795 ) ;
#28567=ORIENTED_EDGE ( 'NONE', *, *, #11218, .F. ) ;
#28574=CARTESIAN_POINT ( 'NONE',  ( -101.4252494179839488, 31.43181965331819683, 32.50001250000000397 ) ) ;
#28579=VERTEX_POINT ( 'NONE', #33496 ) ;
#28589=CARTESIAN_POINT ( 'NONE',  ( 70.80619744048946984, -84.18124734178287838, 32.50000000000000000 ) ) ;
#28591=EDGE_CURVE ( 'NONE', #7201, #4684, #2126, .T. ) ;
#28615=CIRCLE ( 'NONE', #34631, 6.000000000000005329 ) ;
#28618=VECTOR ( 'NONE', #35848, 1000.000000000000000 ) ;
#28621=EDGE_CURVE ( 'NONE', #22736, #5071, #30835, .T. ) ;
#28624=VECTOR ( 'NONE', #34751, 1000.000000000000000 ) ;
#28626=VECTOR ( 'NONE', #22109, 1000.000000000000000 ) ;
#28652=CARTESIAN_POINT ( 'NONE',  ( 90.51363901676214141, -71.13863674840979456, 32.50000000000000711 ) ) ;
#28655=DIRECTION ( 'NONE',  ( 1.000000000000000000, -1.850371707708594366E-15, 0.000000000000000000 ) ) ;
#28687=EDGE_LOOP ( 'NONE', ( #21722, #6103, #36835, #18617 ) ) ;
#28689=AXIS2_PLACEMENT_3D ( 'NONE', #36886, #28429, #31621 ) ;
#28711=LINE ( 'NONE', #2649, #8000 ) ;
#28713=ORIENTED_EDGE ( 'NONE', *, *, #18273, .T. ) ;
#28766=VERTEX_POINT ( 'NONE', #27631 ) ;
#28781=DIRECTION ( 'NONE',  ( 1.000000000000000000, 0.000000000000000000, 0.000000000000000000 ) ) ;
#28784=CARTESIAN_POINT ( 'NONE',  ( 102.5304832720496080, 102.5304832720492527, 27.50000000000000000 ) ) ;
#28796=EDGE_CURVE ( 'NONE', #9908, #3457, #11115, .T. ) ;
#28797=CARTESIAN_POINT ( 'NONE',  ( 55.27226924886129211, 77.26562141134560591, 27.50000000000000000 ) ) ;
#28822=DIRECTION ( 'NONE',  ( 1.000000000000000000, 0.000000000000000000, 0.000000000000000000 ) ) ;
#28830=ORIENTED_EDGE ( 'NONE', *, *, #16688, .T. ) ;
#28858=CARTESIAN_POINT ( 'NONE',  ( -74.30619744048887299, 84.18124734178336155, 32.50000000000000000 ) ) ;
#28859=ORIENTED_EDGE ( 'NONE', *, *, #21482, .F. ) ;
#28880=FACE_OUTER_BOUND ( 'NONE', #29084, .T. ) ;
#28888=EDGE_CURVE ( 'NONE', #20815, #12717, #22764, .T. ) ;
#28891=ADVANCED_FACE ( 'NONE', ( #17119 ), #6774, .F. ) ;
#28924=DIRECTION ( 'NONE',  ( 0.000000000000000000, 0.000000000000000000, 1.000000000000000000 ) ) ;
#28928=ORIENTED_EDGE ( 'NONE', *, *, #20817, .F. ) ;
#28934=CARTESIAN_POINT ( 'NONE',  ( 51.68138994340220904, 113.8157894736842053, 32.50000000000000000 ) ) ;
#28956=CARTESIAN_POINT ( 'NONE',  ( -108.3061974404900241, -19.22934205794863516, 32.50000000000000000 ) ) ;
#28960=ORIENTED_EDGE ( 'NONE', *, *, #29289, .T. ) ;
#28980=CARTESIAN_POINT ( 'NONE',  ( -67.30619744048885877, 84.18124734178336155, 32.50000000000000000 ) ) ;
#28988=ORIENTED_EDGE ( 'NONE', *, *, #7100, .F. ) ;
#28995=CIRCLE ( 'NONE', #2682, 6.000000000000005329 ) ;
#28998=AXIS2_PLACEMENT_3D ( 'NONE', #22061, #25067, #33500 ) ;
#29002=CARTESIAN_POINT ( 'NONE',  ( 110.2237710830536770, 101.7384897088147397, 32.55002500000000509 ) ) ;
#29016=ORIENTED_EDGE ( 'NONE', *, *, #711, .F. ) ;
#29025=VERTEX_POINT ( 'NONE', #412 ) ;
#29026=EDGE_CURVE ( 'NONE', #3457, #9908, #12934, .T. ) ;
#29037=CARTESIAN_POINT ( 'NONE',  ( 88.66518046043564993, 71.67709580616666187, 32.50000000000000000 ) ) ;
#29045=ORIENTED_EDGE ( 'NONE', *, *, #12293, .F. ) ;
#29051=VECTOR ( 'NONE', #31703, 1000.000000000000000 ) ;
#29073=CARTESIAN_POINT ( 'NONE',  ( 98.28784258492957804, -106.7731239591692116, 27.50000000000000000 ) ) ;
#29084=EDGE_LOOP ( 'NONE', ( #30927, #2571, #21786, #18602, #24802, #29703, #27712, #26358, #6359, #24120, #22183, #17472, #46, #33690, #13128, #16732, #22054, #5049, #17170, #9933, #13183, #32033, #30041, #13892, #9182, #28241, #28494, #33750, #21739, #20459, #30177, #1880, #16559, #33252, #13896 ) ) ;
#29087=CARTESIAN_POINT ( 'NONE',  ( -149.8799519615615736, 6.000000000001555200, 32.55002500000000509 ) ) ;
#29088=CARTESIAN_POINT ( 'NONE',  ( 5.999999999999985789, 149.8799519615616305, 27.50000000000000000 ) ) ;
#29100=CIRCLE ( 'NONE', #2786, 30.00000000000000000 ) ;
#29135=FACE_OUTER_BOUND ( 'NONE', #9053, .T. ) ;
#29146=DIRECTION ( 'NONE',  ( 0.000000000000000000, -0.000000000000000000, -1.000000000000000000 ) ) ;
#29159=ORIENTED_EDGE ( 'NONE', *, *, #36790, .T. ) ;
#29164=ORIENTED_EDGE ( 'NONE', *, *, #27520, .F. ) ;
#29168=CIRCLE ( 'NONE', #2818, 3.500000000000003109 ) ;
#29172=ORIENTED_EDGE ( 'NONE', *, *, #22141, .T. ) ;
#29201=DIRECTION ( 'NONE',  ( 0.000000000000000000, 0.000000000000000000, 1.000000000000000000 ) ) ;
#29232=ORIENTED_EDGE ( 'NONE', *, *, #34712, .F. ) ;
#29243=ORIENTED_EDGE ( 'NONE', *, *, #3206, .F. ) ;
#29254=ORIENTED_EDGE ( 'NONE', *, *, #1950, .F. ) ;
#29274=ORIENTED_EDGE ( 'NONE', *, *, #16539, .T. ) ;
#29278=CARTESIAN_POINT ( 'NONE',  ( -104.3561661892587722, 35.61482833294783745, 32.49999999999999289 ) ) ;
#29289=EDGE_CURVE ( 'NONE', #31753, #8057, #20721, .T. ) ;
#29292=EDGE_CURVE ( 'NONE', #8890, #33391, #8456, .T. ) ;
#29301=VECTOR ( 'NONE', #12090, 1000.000000000000000 ) ;
#29316=LINE ( 'NONE', #26495, #26745 ) ;
#29329=VERTEX_POINT ( 'NONE', #9366 ) ;
#29340=DIRECTION ( 'NONE',  ( -1.000000000000000000, 0.000000000000000000, 0.000000000000000000 ) ) ;
#29343=EDGE_LOOP ( 'NONE', ( #14052, #25933, #33194, #28567 ) ) ;
#29349=EDGE_CURVE ( 'NONE', #35112, #35608, #18353, .T. ) ;
#29351=ORIENTED_EDGE ( 'NONE', *, *, #24453, .F. ) ;
#29355=LINE ( 'NONE', #26174, #21846 ) ;
#29356=ADVANCED_FACE ( 'NONE', ( #3571 ), #6367, .F. ) ;
#29357=EDGE_CURVE ( 'NONE', #31244, #22880, #16538, .T. ) ;
#29361=EDGE_LOOP ( 'NONE', ( #1973, #7375, #12077, #27447 ) ) ;
#29363=ADVANCED_FACE ( 'NONE', ( #11985 ), #23614, .T. ) ;
#29365=ORIENTED_EDGE ( 'NONE', *, *, #15104, .T. ) ;
#29380=CARTESIAN_POINT ( 'NONE',  ( -149.8799519615616873, -5.999999999998430589, 32.50000000000000000 ) ) ;
#29393=EDGE_CURVE ( 'NONE', #4570, #27930, #29424, .T. ) ;
#29399=EDGE_CURVE ( 'NONE', #4461, #10948, #6736, .T. ) ;
#29403=ORIENTED_EDGE ( 'NONE', *, *, #4659, .T. ) ;
#29424=LINE ( 'NONE', #28858, #13588 ) ;
#29430=CYLINDRICAL_SURFACE ( 'NONE', #19647, 30.00000000000000000 ) ;
#29440=FACE_BOUND ( 'NONE', #27139, .T. ) ;
#29443=VECTOR ( 'NONE', #13361, 1000.000000000000000 ) ;
#29457=CARTESIAN_POINT ( 'NONE',  ( 104.8061974404898820, 19.22934205794938478, 32.50000000000000000 ) ) ;
#29474=DIRECTION ( 'NONE',  ( -0.000000000000000000, -0.000000000000000000, 1.000000000000000000 ) ) ;
#29481=CARTESIAN_POINT ( 'NONE',  ( -17.74171217315199200, -112.6247319038655235, 32.50000000000000711 ) ) ;
#29495=DIRECTION ( 'NONE',  ( 0.000000000000000000, 0.000000000000000000, 1.000000000000000000 ) ) ;
#29510=CARTESIAN_POINT ( 'NONE',  ( 145.0000000000000568, -5.056524707326808249E-13, 32.55002500000000509 ) ) ;
#29515=DIRECTION ( 'NONE',  ( -0.000000000000000000, -0.000000000000000000, 1.000000000000000000 ) ) ;
#29516=DIRECTION ( 'NONE',  ( -3.554796214472773777E-16, -1.000000000000000000, 0.000000000000000000 ) ) ;
#29533=LINE ( 'NONE', #18292, #10159 ) ;
#29537=ORIENTED_EDGE ( 'NONE', *, *, #22651, .F. ) ;
#29538=DIRECTION ( 'NONE',  ( 0.000000000000000000, -1.000000000000000000, 0.000000000000000000 ) ) ;
#29548=ORIENTED_EDGE ( 'NONE', *, *, #30284, .T. ) ;
#29564=CARTESIAN_POINT ( 'NONE',  ( 106.7731239591688848, 98.28784258492994752, 32.50000000000000000 ) ) ;
#29571=ORIENTED_EDGE ( 'NONE', *, *, #6303, .F. ) ;
#29582=EDGE_LOOP ( 'NONE', ( #12406, #33171 ) ) ;
#29583=ADVANCED_BREP_SHAPE_REPRESENTATION ( '', ( #32134, #21385 ), #25533 ) ;
#29584=EDGE_CURVE ( 'NONE', #4310, #33855, #21378, .T. ) ;
#29592=DIRECTION ( 'NONE',  ( 0.000000000000000000, -0.000000000000000000, -1.000000000000000000 ) ) ;
#29594=ADVANCED_FACE ( 'NONE', ( #19668 ), #17530, .F. ) ;
#29595=FACE_OUTER_BOUND ( 'NONE', #16741, .T. ) ;
#29598=CARTESIAN_POINT ( 'NONE',  ( 101.4252628994511980, 31.43180897937319784, 32.50001250000000397 ) ) ;
#29599=DIRECTION ( 'NONE',  ( -0.000000000000000000, -0.000000000000000000, 1.000000000000000000 ) ) ;
#29627=VECTOR ( 'NONE', #29538, 1000.000000000000000 ) ;
#29656=CIRCLE ( 'NONE', #15894, 3.500000000000003109 ) ;
#29659=ORIENTED_EDGE ( 'NONE', *, *, #19618, .T. ) ;
#29662=AXIS2_PLACEMENT_3D ( 'NONE', #34180, #8648, #14468 ) ;
#29664=EDGE_CURVE ( 'NONE', #27343, #32462, #31099, .T. ) ;
#29690=STYLED_ITEM ( 'NONE', ( #31470 ), #29583 ) ;
#29693=CIRCLE ( 'NONE', #24332, 6.000000000000005329 ) ;
#29697=FACE_OUTER_BOUND ( 'NONE', #19173, .T. ) ;
#29703=ORIENTED_EDGE ( 'NONE', *, *, #9812, .F. ) ;
#29713=AXIS2_PLACEMENT_3D ( 'NONE', #11605, #26608, #739 ) ;
#29716=LINE ( 'NONE', #3849, #22737 ) ;
#29720=AXIS2_PLACEMENT_3D ( 'NONE', #1786, #33085, #4958 ) ;
#29722=CIRCLE ( 'NONE', #17187, 3.500000000000003109 ) ;
#29745=FACE_OUTER_BOUND ( 'NONE', #17507, .T. ) ;
#29754=FACE_OUTER_BOUND ( 'NONE', #684, .T. ) ;
#29756=CARTESIAN_POINT ( 'NONE',  ( -106.7731239591695669, -98.28784258492920856, 32.50000000000000000 ) ) ;
#29757=ORIENTED_EDGE ( 'NONE', *, *, #31974, .T. ) ;
#29764=VECTOR ( 'NONE', #21812, 1000.000000000000000 ) ;
#29782=ORIENTED_EDGE ( 'NONE', *, *, #28216, .F. ) ;
#29783=AXIS2_PLACEMENT_3D ( 'NONE', #3866, #8953, #14754 ) ;
#29804=CARTESIAN_POINT ( 'NONE',  ( 102.5304832720496080, 102.5304832720492527, 32.50000000000000000 ) ) ;
#29805=ORIENTED_EDGE ( 'NONE', *, *, #4738, .F. ) ;
#29810=ORIENTED_EDGE ( 'NONE', *, *, #5029, .F. ) ;
#29816=CARTESIAN_POINT ( 'NONE',  ( 70.80619744048946984, -84.18124734178287838, 32.50000000000000000 ) ) ;
#29818=AXIS2_PLACEMENT_3D ( 'NONE', #13611, #19422, #5178 ) ;
#29823=ADVANCED_FACE ( 'NONE', ( #12456 ), #35173, .T. ) ;
#29826=EDGE_CURVE ( 'NONE', #33879, #24561, #23790, .T. ) ;
#29830=ORIENTED_EDGE ( 'NONE', *, *, #9460, .F. ) ;
#29840=CARTESIAN_POINT ( 'NONE',  ( -6.123233995736731770E-16, 145.0000000000000568, 32.55002500000000509 ) ) ;
#29849=CARTESIAN_POINT ( 'NONE',  ( 108.3061974404897825, -19.22934205795014151, 32.50000000000000000 ) ) ;
#29850=VECTOR ( 'NONE', #31668, 1000.000000000000000 ) ;
#29852=ORIENTED_EDGE ( 'NONE', *, *, #4764, .F. ) ;
#29862=CARTESIAN_POINT ( 'NONE',  ( -6.000000000000000000, 145.0000000000000568, 32.50000000000000000 ) ) ;
#29890=CARTESIAN_POINT ( 'NONE',  ( -51.68138994340220904, 113.8157894736842053, 32.50000000000000000 ) ) ;
#29895=EDGE_CURVE ( 'NONE', #35112, #13025, #19223, .T. ) ;
#29906=ORIENTED_EDGE ( 'NONE', *, *, #36925, .F. ) ;
#29916=DIRECTION ( 'NONE',  ( 3.554796214472773777E-16, 1.000000000000000000, -0.000000000000000000 ) ) ;
#29933=DIRECTION ( 'NONE',  ( 0.000000000000000000, 0.000000000000000000, 1.000000000000000000 ) ) ;
#29964=CARTESIAN_POINT ( 'NONE',  ( -98.28784258492883907, 106.7731239591698937, 27.50000000000000000 ) ) ;
#29973=CARTESIAN_POINT ( 'NONE',  ( 106.7731239591688848, 98.28784258492994752, 32.55002500000000509 ) ) ;
#30040=CARTESIAN_POINT ( 'NONE',  ( 124.4080600076931375, 12.15049814296589226, 32.50000000000000000 ) ) ;
#30041=ORIENTED_EDGE ( 'NONE', *, *, #9671, .F. ) ;
#30063=DIRECTION ( 'NONE',  ( 1.000000000000000000, 0.000000000000000000, 0.000000000000000000 ) ) ;
#30067=DIRECTION ( 'NONE',  ( 0.000000000000000000, -0.000000000000000000, -1.000000000000000000 ) ) ;
#30077=EDGE_LOOP ( 'NONE', ( #130, #30328 ) ) ;
#30094=CARTESIAN_POINT ( 'NONE',  ( 0.000000000000000000, 0.000000000000000000, 27.50000000000000000 ) ) ;
#30098=DIRECTION ( 'NONE',  ( 0.000000000000000000, 0.000000000000000000, 1.000000000000000000 ) ) ;
#30100=CARTESIAN_POINT ( 'NONE',  ( 23.49154088336464241, 103.5526315789473699, 32.50000000000000000 ) ) ;
#30102=DIRECTION ( 'NONE',  ( -0.7071067811865514585, -0.7071067811865435759, 0.000000000000000000 ) ) ;
#30149=VERTEX_POINT ( 'NONE', #23116 ) ;
#30153=VERTEX_POINT ( 'NONE', #34570 ) ;
#30167=CARTESIAN_POINT ( 'NONE',  ( 102.9785387920993003, -33.47425447865018810, 32.49999999999999289 ) ) ;
#30173=ADVANCED_FACE ( 'NONE', ( #22568 ), #25573, .T. ) ;
#30177=ORIENTED_EDGE ( 'NONE', *, *, #23387, .F. ) ;
#30225=CIRCLE ( 'NONE', #14059, 6.000000000000005329 ) ;
#30237=DIRECTION ( 'NONE',  ( -1.000000000000000000, 0.000000000000000000, 0.000000000000000000 ) ) ;
#30243=CARTESIAN_POINT ( 'NONE',  ( -74.30619744049063513, -84.18124734178186941, 32.50000000000000000 ) ) ;
#30264=CIRCLE ( 'NONE', #17098, 3.500000000000003109 ) ;
#30272=CIRCLE ( 'NONE', #23692, 30.00000000000000000 ) ;
#30273=VECTOR ( 'NONE', #24698, 1000.000000000000000 ) ;
#30284=EDGE_CURVE ( 'NONE', #16882, #37014, #26664, .T. ) ;
#30291=AXIS2_PLACEMENT_3D ( 'NONE', #14410, #25849, #17410 ) ;
#30295=AXIS2_PLACEMENT_3D ( 'NONE', #22772, #25574, #13937 ) ;
#30328=ORIENTED_EDGE ( 'NONE', *, *, #3208, .T. ) ;
#30331=ORIENTED_EDGE ( 'NONE', *, *, #29026, .T. ) ;
#30342=CARTESIAN_POINT ( 'NONE',  ( 40.99999999999999289, 103.4105893997321743, 32.50000000000000000 ) ) ;
#30384=DIRECTION ( 'NONE',  ( 0.000000000000000000, 0.000000000000000000, 1.000000000000000000 ) ) ;
#30387=CIRCLE ( 'NONE', #15430, 30.00000000000000000 ) ;
#30403=EDGE_LOOP ( 'NONE', ( #16809, #17921, #23580, #17770 ) ) ;
#30408=CYLINDRICAL_SURFACE ( 'NONE', #15204, 3.499999999999996003 ) ;
#30430=CARTESIAN_POINT ( 'NONE',  ( -4.242640687119211051, 4.242640687119288323, 32.50000000000000000 ) ) ;
#30440=CIRCLE ( 'NONE', #35248, 3.500000000000003109 ) ;
#30454=DIRECTION ( 'NONE',  ( 0.000000000000000000, 0.000000000000000000, 1.000000000000000000 ) ) ;
#30470=CARTESIAN_POINT ( 'NONE',  ( -5.999999999999947597, 2.132877728683645235E-15, 32.50000000000000000 ) ) ;
#30481=EDGE_CURVE ( 'NONE', #24583, #7532, #14263, .T. ) ;
#30494=ORIENTED_EDGE ( 'NONE', *, *, #33765, .F. ) ;
#30501=CARTESIAN_POINT ( 'NONE',  ( 0.000000000000000000, 0.000000000000000000, 27.50000000000000000 ) ) ;
#30506=ORIENTED_EDGE ( 'NONE', *, *, #33023, .F. ) ;
#30516=CARTESIAN_POINT ( 'NONE',  ( 145.0000000000000284, -6.000000000000504485, 32.55002500000000509 ) ) ;
#30522=CARTESIAN_POINT ( 'NONE',  ( -106.8619802314695306, 52.03961299853113331, 32.50000000000000000 ) ) ;
#30539=CARTESIAN_POINT ( 'NONE',  ( -6.123233995736731770E-16, 145.0000000000000568, 32.50000000000000000 ) ) ;
#30543=CARTESIAN_POINT ( 'NONE',  ( -101.8947913453489349, 31.99226454438814571, 32.50000000000000711 ) ) ;
#30548=ORIENTED_EDGE ( 'NONE', *, *, #22476, .F. ) ;
#30563=DIRECTION ( 'NONE',  ( -0.000000000000000000, -0.000000000000000000, -1.000000000000000000 ) ) ;
#30567=( NAMED_UNIT ( * ) PLANE_ANGLE_UNIT ( ) SI_UNIT ( $, .RADIAN. ) );
#30599=DIRECTION ( 'NONE',  ( 1.000000000000000000, 0.000000000000000000, 0.000000000000000000 ) ) ;
#30601=VERTEX_POINT ( 'NONE', #20266 ) ;
#30610=LINE ( 'NONE', #11294, #1026 ) ;
#30623=VERTEX_POINT ( 'NONE', #8462 ) ;
#30630=CARTESIAN_POINT ( 'NONE',  ( 18.28331374579376956, 112.2394282457694459, 27.49998799999999832 ) ) ;
#30641=DIRECTION ( 'NONE',  ( 1.000000000000000000, 0.000000000000000000, 0.000000000000000000 ) ) ;
#30649=FACE_BOUND ( 'NONE', #30077, .T. ) ;
#30656=ADVANCED_FACE ( 'NONE', ( #14820 ), #29430, .T. ) ;
#30663=VERTEX_POINT ( 'NONE', #3749 ) ;
#30672=ORIENTED_EDGE ( 'NONE', *, *, #3019, .F. ) ;
#30695=B_SPLINE_CURVE_WITH_KNOTS ( 'NONE', 3,
 ( #18914, #30543, #16293, #32069, #29278, #15035, #26461, #21720, #35101, #1667, #13104, #32981 ),
 .UNSPECIFIED., .F., .F.,
 ( 4, 2, 1, 2, 2, 1, 4 ),
 ( 0.05563282717590184445, 0.06951991305345063543, 0.08340699893099942641, 0.1111811706860971471, 0.1250682565636460630, 0.1389553424411949512, 0.1667295141962928384 ),
 .UNSPECIFIED. ) ;
#30729=FILL_AREA_STYLE_COLOUR ( '', #33864 ) ;
#30774=CARTESIAN_POINT ( 'NONE',  ( -106.6136243914056507, -41.75127244461555875, 32.50000000000000000 ) ) ;
#30778=AXIS2_PLACEMENT_3D ( 'NONE', #29804, #1305, #27364 ) ;
#30788=DIRECTION ( 'NONE',  ( -0.000000000000000000, 1.000000000000000000, 0.000000000000000000 ) ) ;
#30811=ORIENTED_EDGE ( 'NONE', *, *, #21128, .F. ) ;
#30821=CARTESIAN_POINT ( 'NONE',  ( 23.02815535700703364, -104.7522195559561595, 32.49999999999999289 ) ) ;
#30830=CARTESIAN_POINT ( 'NONE',  ( -98.28784258492883907, 106.7731239591698937, 32.55002500000000509 ) ) ;
#30835=CIRCLE ( 'NONE', #2718, 30.00000000000000000 ) ;
#30847=EDGE_CURVE ( 'NONE', #17078, #37014, #4137, .T. ) ;
#30854=CARTESIAN_POINT ( 'NONE',  ( -6.000000000000000000, 149.8799519615616305, 32.55002500000000509 ) ) ;
#30867=DIRECTION ( 'NONE',  ( 0.000000000000000000, 0.000000000000000000, 1.000000000000000000 ) ) ;
#30887=DIRECTION ( 'NONE',  ( -0.000000000000000000, -0.000000000000000000, 1.000000000000000000 ) ) ;
#30902=VECTOR ( 'NONE', #17568, 1000.000000000000000 ) ;
#30908=CARTESIAN_POINT ( 'NONE',  ( -93.06171781654443009, -70.18599611865349175, 32.50000000000000000 ) ) ;
#30927=ORIENTED_EDGE ( 'NONE', *, *, #19394, .F. ) ;
#30935=EDGE_CURVE ( 'NONE', #1224, #1952, #41, .T. ) ;
#30943=DIRECTION ( 'NONE',  ( 0.000000000000000000, 0.000000000000000000, 1.000000000000000000 ) ) ;
#30951=VECTOR ( 'NONE', #12754, 999.9999999999998863 ) ;
#30956=ORIENTED_EDGE ( 'NONE', *, *, #19168, .T. ) ;
#30970=DIRECTION ( 'NONE',  ( 1.000000000000000000, 0.000000000000000000, 0.000000000000000000 ) ) ;
#30993=VECTOR ( 'NONE', #30563, 1000.000000000000000 ) ;
#31014=VECTOR ( 'NONE', #18309, 1000.000000000000000 ) ;
#31027=CARTESIAN_POINT ( 'NONE',  ( 19.04456692557281983, -111.2113061358873836, 32.49999999999999289 ) ) ;
#31067=EDGE_LOOP ( 'NONE', ( #19843, #12866, #19862, #24940 ) ) ;
#31072=AXIS2_PLACEMENT_3D ( 'NONE', #31908, #6075, #34390 ) ;
#31084=AXIS2_PLACEMENT_3D ( 'NONE', #8761, #22838, #25835 ) ;
#31087=EDGE_LOOP ( 'NONE', ( #26071, #13333, #9197, #34792, #12462, #5367, #26582, #19509, #18191, #2244, #32954, #33437, #839, #14508, #17843, #13957, #24486, #29164, #9616, #14588, #1784, #32230, #4210, #10291, #21110, #5619, #3, #24152, #12648 ) ) ;
#31091=LINE ( 'NONE', #5225, #5248 ) ;
#31096=AXIS2_PLACEMENT_3D ( 'NONE', #10233, #10045, #21280 ) ;
#31099=LINE ( 'NONE', #16474, #36930 ) ;
#31126=VECTOR ( 'NONE', #79, 1000.000000000000000 ) ;
#31129=AXIS2_PLACEMENT_3D ( 'NONE', #7143, #12363, #23632 ) ;
#31164=VERTEX_POINT ( 'NONE', #20959 ) ;
#31169=VERTEX_POINT ( 'NONE', #525 ) ;
#31173=ORIENTED_EDGE ( 'NONE', *, *, #13306, .T. ) ;
#31183=CARTESIAN_POINT ( 'NONE',  ( -6.284666409917640040E-14, -6.000000000000000000, 32.50000000000000000 ) ) ;
#31193=CARTESIAN_POINT ( 'NONE',  ( 22.62085438525362591, 105.9441488773368860, 27.49998799999998411 ) ) ;
#31194=LINE ( 'NONE', #5509, #19364 ) ;
#31202=ORIENTED_EDGE ( 'NONE', *, *, #19624, .T. ) ;
#31222=EDGE_CURVE ( 'NONE', #19410, #10608, #15701, .T. ) ;
#31244=VERTEX_POINT ( 'NONE', #13069 ) ;
#31253=ORIENTED_EDGE ( 'NONE', *, *, #21145, .F. ) ;
#31259=EDGE_LOOP ( 'NONE', ( #24079, #8962 ) ) ;
#31264=ORIENTED_EDGE ( 'NONE', *, *, #3313, .F. ) ;
#31272=CARTESIAN_POINT ( 'NONE',  ( -107.0107436789505329, -51.13647734612944618, 32.50000000000000711 ) ) ;
#31290=ORIENTED_EDGE ( 'NONE', *, *, #28320, .F. ) ;
#31309=CARTESIAN_POINT ( 'NONE',  ( 0.000000000000000000, 0.000000000000000000, 32.50000000000000000 ) ) ;
#31318=CARTESIAN_POINT ( 'NONE',  ( -4.242640687119273224, -4.242640687119226151, 27.50000000000000000 ) ) ;
#31329=DIRECTION ( 'NONE',  ( 1.000000000000000000, 0.000000000000000000, 0.000000000000000000 ) ) ;
#31338=AXIS2_PLACEMENT_3D ( 'NONE', #9048, #28362, #8870 ) ;
#31370=CARTESIAN_POINT ( 'NONE',  ( -40.99999999999999289, 103.4105893997321743, 32.50000000000000000 ) ) ;
#31378=ORIENTED_EDGE ( 'NONE', *, *, #35594, .F. ) ;
#31419=VECTOR ( 'NONE', #20927, 1000.000000000000000 ) ;
#31429=CARTESIAN_POINT ( 'NONE',  ( 98.28784258493033121, 106.7731239591685437, 32.55002500000000509 ) ) ;
#31437=DIRECTION ( 'NONE',  ( 1.000000000000000000, 0.000000000000000000, 0.000000000000000000 ) ) ;
#31444=VECTOR ( 'NONE', #8759, 1000.000000000000000 ) ;
#31445=EDGE_LOOP ( 'NONE', ( #27493, #15232, #5517, #33155 ) ) ;
#31452=DIRECTION ( 'NONE',  ( -0.000000000000000000, -0.000000000000000000, -1.000000000000000000 ) ) ;
#31459=CARTESIAN_POINT ( 'NONE',  ( -149.8799519615616873, -5.999999999998430589, 32.55002500000000509 ) ) ;
#31470=PRESENTATION_STYLE_ASSIGNMENT (( #17252 ) ) ;
#31472=AXIS2_PLACEMENT_3D ( 'NONE', #31725, #9609, #20850 ) ;
#31480=ADVANCED_FACE ( 'NONE', ( #31948 ), #843, .F. ) ;
#31541=CIRCLE ( 'NONE', #15390, 3.499999999999996003 ) ;
#31559=CYLINDRICAL_SURFACE ( 'NONE', #36494, 30.00000000000000000 ) ;
#31577=DIRECTION ( 'NONE',  ( 1.000000000000000000, 0.000000000000000000, 0.000000000000000000 ) ) ;
#31585=ORIENTED_EDGE ( 'NONE', *, *, #3233, .F. ) ;
#31598=CARTESIAN_POINT ( 'NONE',  ( -70.80619744049063513, -84.18124734178186941, 32.50000000000000000 ) ) ;
#31607=VECTOR ( 'NONE', #22608, 1000.000000000000000 ) ;
#31621=DIRECTION ( 'NONE',  ( 1.000000000000000000, 0.000000000000000000, 0.000000000000000000 ) ) ;
#31648=DIRECTION ( 'NONE',  ( 1.000000000000000000, 0.000000000000000000, 0.000000000000000000 ) ) ;
#31650=DIRECTION ( 'NONE',  ( 1.000000000000000000, 0.000000000000000000, 0.000000000000000000 ) ) ;
#31668=DIRECTION ( 'NONE',  ( -0.000000000000000000, -0.000000000000000000, -1.000000000000000000 ) ) ;
#31688=CIRCLE ( 'NONE', #11934, 30.00000000000000000 ) ;
#31692=CIRCLE ( 'NONE', #14340, 6.000000000000005329 ) ;
#31696=CARTESIAN_POINT ( 'NONE',  ( -145.0000000000001137, -5.999999999998481215, 27.50000000000000000 ) ) ;
#31703=DIRECTION ( 'NONE',  ( 0.000000000000000000, -1.000000000000000000, 0.000000000000000000 ) ) ;
#31712=AXIS2_PLACEMENT_3D ( 'NONE', #34059, #5543, #8908 ) ;
#31725=CARTESIAN_POINT ( 'NONE',  ( -106.7731239591695669, -98.28784258492920856, 32.55002500000000509 ) ) ;
#31727=DIRECTION ( 'NONE',  ( 1.000000000000000000, 0.000000000000000000, 0.000000000000000000 ) ) ;
#31734=AXIS2_PLACEMENT_3D ( 'NONE', #735, #18366, #15361 ) ;
#31739=AXIS2_PLACEMENT_3D ( 'NONE', #31989, #14970, #6705 ) ;
#31748=CARTESIAN_POINT ( 'NONE',  ( -23.02818743869751827, -104.7521194859946263, 32.50000000000001421 ) ) ;
#31750=VERTEX_POINT ( 'NONE', #375 ) ;
#31753=VERTEX_POINT ( 'NONE', #31696 ) ;
#31771=DIRECTION ( 'NONE',  ( -0.000000000000000000, -0.000000000000000000, -1.000000000000000000 ) ) ;
#31788=ADVANCED_FACE ( 'NONE', ( #28325 ), #2646, .F. ) ;
#31806=VERTEX_POINT ( 'NONE', #19896 ) ;
#31815=DIRECTION ( 'NONE',  ( 1.000000000000000000, 0.000000000000000000, 0.000000000000000000 ) ) ;
#31842=CARTESIAN_POINT ( 'NONE',  ( 106.9296898191251159, 51.67694400691266310, 32.49999999999999289 ) ) ;
#31850=CARTESIAN_POINT ( 'NONE',  ( 23.49154088336464241, -103.5526315789473699, 27.50000000000000000 ) ) ;
#31883=ORIENTED_EDGE ( 'NONE', *, *, #30481, .F. ) ;
#31902=ORIENTED_EDGE ( 'NONE', *, *, #4650, .T. ) ;
#31908=CARTESIAN_POINT ( 'NONE',  ( -82.27241335952211898, -47.49999999999924682, 27.50000000000000000 ) ) ;
#31930=LINE ( 'NONE', #12064, #8863 ) ;
#31941=DIRECTION ( 'NONE',  ( 1.000000000000000000, 0.000000000000000000, 0.000000000000000000 ) ) ;
#31948=FACE_OUTER_BOUND ( 'NONE', #30403, .T. ) ;
#31965=DIRECTION ( 'NONE',  ( 1.000000000000000000, 0.000000000000000000, 0.000000000000000000 ) ) ;
#31967=DIRECTION ( 'NONE',  ( 1.000000000000000000, -1.047444401652940007E-14, 0.000000000000000000 ) ) ;
#31974=EDGE_CURVE ( 'NONE', #35726, #36154, #938, .T. ) ;
#31987=CARTESIAN_POINT ( 'NONE',  ( -107.2742747693529566, -47.50000423952285900, 32.50001250000000397 ) ) ;
#31989=CARTESIAN_POINT ( 'NONE',  ( -37.50000000000000000, -103.4105893997321743, 27.50000000000000000 ) ) ;
#31990=ORIENTED_EDGE ( 'NONE', *, *, #19162, .T. ) ;
#31991=ORIENTED_EDGE ( 'NONE', *, *, #2709, .T. ) ;
#32003=FACE_OUTER_BOUND ( 'NONE', #3269, .T. ) ;
#32004=EDGE_LOOP ( 'NONE', ( #19183, #12433, #13787, #16723 ) ) ;
#32007=EDGE_CURVE ( 'NONE', #9234, #30623, #16314, .T. ) ;
#32010=DIRECTION ( 'NONE',  ( 1.000000000000000000, 0.000000000000000000, 0.000000000000000000 ) ) ;
#32013=ORIENTED_EDGE ( 'NONE', *, *, #22, .T. ) ;
#32023=DIRECTION ( 'NONE',  ( 1.000000000000000000, 0.000000000000000000, 0.000000000000000000 ) ) ;
#32024=CARTESIAN_POINT ( 'NONE',  ( 107.1113515669819236, 50.40365827702301260, 32.50000000000000711 ) ) ;
#32032=CARTESIAN_POINT ( 'NONE',  ( -70.80619744049063513, -84.18124734178186941, 27.50000000000000000 ) ) ;
#32033=ORIENTED_EDGE ( 'NONE', *, *, #18304, .T. ) ;
#32044=VERTEX_POINT ( 'NONE', #24186 ) ;
#32046=DIRECTION ( 'NONE',  ( 1.000000000000000000, 0.000000000000000000, -0.000000000000000000 ) ) ;
#32055=CIRCLE ( 'NONE', #11122, 6.000000000000005329 ) ;
#32069=CARTESIAN_POINT ( 'NONE',  ( -103.1837242358309510, 33.77655254667255491, 32.50000000000000000 ) ) ;
#32071=CARTESIAN_POINT ( 'NONE',  ( 111.8061974404897825, -19.22934205795014151, 32.50000000000000000 ) ) ;
#32079=ORIENTED_EDGE ( 'NONE', *, *, #23414, .T. ) ;
#32080=CARTESIAN_POINT ( 'NONE',  ( -98.28784258493107018, -106.7731239591678616, 27.50000000000000000 ) ) ;
#32087=EDGE_CURVE ( 'NONE', #16622, #26755, #6283, .T. ) ;
#32093=VECTOR ( 'NONE', #1760, 1000.000000000000000 ) ;
#32098=ORIENTED_EDGE ( 'NONE', *, *, #23714, .T. ) ;
#32103=ORIENTED_EDGE ( 'NONE', *, *, #22851, .T. ) ;
#32107=CYLINDRICAL_SURFACE ( 'NONE', #4214, 150.0000000000000284 ) ;
#32120=DIRECTION ( 'NONE',  ( 1.000000000000000000, 0.000000000000000000, 0.000000000000000000 ) ) ;
#32134=MANIFOLD_SOLID_BREP ( 'CirPattern3', #11775 ) ;
#32153=DIRECTION ( 'NONE',  ( 0.000000000000000000, 0.000000000000000000, 1.000000000000000000 ) ) ;
#32167=AXIS2_PLACEMENT_3D ( 'NONE', #3446, #28924, #14677 ) ;
#32170=DIRECTION ( 'NONE',  ( 1.000000000000000000, 0.000000000000000000, 0.000000000000000000 ) ) ;
#32182=AXIS2_PLACEMENT_3D ( 'NONE', #19229, #1400, #30641 ) ;
#32185=EDGE_LOOP ( 'NONE', ( #29254, #2184 ) ) ;
#32192=ORIENTED_EDGE ( 'NONE', *, *, #36022, .F. ) ;
#32230=ORIENTED_EDGE ( 'NONE', *, *, #12830, .T. ) ;
#32236=CARTESIAN_POINT ( 'NONE',  ( 0.000000000000000000, 0.000000000000000000, 27.50000000000000000 ) ) ;
#32279=AXIS2_PLACEMENT_3D ( 'NONE', #25243, #16811, #36671 ) ;
#32312=CARTESIAN_POINT ( 'NONE',  ( -104.8061974404900241, -19.22934205794863516, 32.50000000000000000 ) ) ;
#32315=LINE ( 'NONE', #9243, #6961 ) ;
#32340=CIRCLE ( 'NONE', #31739, 3.499999999999996003 ) ;
#32418=CARTESIAN_POINT ( 'NONE',  ( 0.000000000000000000, 0.000000000000000000, 32.50000000000000000 ) ) ;
#32422=CARTESIAN_POINT ( 'NONE',  ( 78.56331849833966885, 72.23155790780543839, 32.50000000000000000 ) ) ;
#32423=CARTESIAN_POINT ( 'NONE',  ( -51.68138994340220904, 113.8157894736842053, 32.50000000000000000 ) ) ;
#32440=LINE ( 'NONE', #26445, #26341 ) ;
#32462=VERTEX_POINT ( 'NONE', #16273 ) ;
#32474=ORIENTED_EDGE ( 'NONE', *, *, #22141, .F. ) ;
#32482=FACE_OUTER_BOUND ( 'NONE', #4773, .T. ) ;
#32483=CIRCLE ( 'NONE', #17500, 25.00000000000000000 ) ;
#32492=DIRECTION ( 'NONE',  ( 1.000000000000000000, 0.000000000000000000, 0.000000000000000000 ) ) ;
#32496=CARTESIAN_POINT ( 'NONE',  ( -108.3061974404896262, 19.22934205795090534, 32.50000000000000000 ) ) ;
#32497=EDGE_CURVE ( 'NONE', #20832, #16892, #21699, .T. ) ;
#32517=ORIENTED_EDGE ( 'NONE', *, *, #29399, .T. ) ;
#32529=FACE_OUTER_BOUND ( 'NONE', #12590, .T. ) ;
#32552=ADVANCED_FACE ( 'NONE', ( #7841 ), #22825, .F. ) ;
#32557=CARTESIAN_POINT ( 'NONE',  ( -55.27226924886182502, -77.26562141134519379, 27.50000000000000000 ) ) ;
#32600=CARTESIAN_POINT ( 'NONE',  ( 107.2802272138360422, 45.32406911912114822, 32.50000000000000000 ) ) ;
#32620=VERTEX_POINT ( 'NONE', #11906 ) ;
#32630=CIRCLE ( 'NONE', #21262, 3.500000000000003109 ) ;
#32633=CIRCLE ( 'NONE', #11065, 3.499999999999996003 ) ;
#32675=EDGE_CURVE ( 'NONE', #33391, #6042, #30264, .T. ) ;
#32693=DIRECTION ( 'NONE',  ( 0.000000000000000000, 0.000000000000000000, 1.000000000000000000 ) ) ;
#32694=LINE ( 'NONE', #18651, #17805 ) ;
#32695=CARTESIAN_POINT ( 'NONE',  ( 5.999999999999985789, 149.8799519615616305, 32.50000000000000000 ) ) ;
#32697=AXIS2_PLACEMENT_3D ( 'NONE', #12568, #12737, #24023 ) ;
#32723=FACE_BOUND ( 'NONE', #2692, .T. ) ;
#32732=LINE ( 'NONE', #23946, #29301 ) ;
#32737=AXIS2_PLACEMENT_3D ( 'NONE', #11632, #23284, #17467 ) ;
#32751=ORIENTED_EDGE ( 'NONE', *, *, #20100, .F. ) ;
#32755=AXIS2_PLACEMENT_3D ( 'NONE', #28934, #9455, #20886 ) ;
#32765=CARTESIAN_POINT ( 'NONE',  ( -93.06207005441154934, 70.18581618242465936, 32.50000000000000000 ) ) ;
#32771=DIRECTION ( 'NONE',  ( -1.000000000000000000, 0.000000000000000000, 0.000000000000000000 ) ) ;
#32772=ORIENTED_EDGE ( 'NONE', *, *, #22923, .F. ) ;
#32786=COLOUR_RGB ( '', 0.66274510, 0.83137255, 0.94901961) ;
#32797=ORIENTED_EDGE ( 'NONE', *, *, #4650, .F. ) ;
#32866=AXIS2_PLACEMENT_3D ( 'NONE', #15063, #20877, #26489 ) ;
#32886=VERTEX_POINT ( 'NONE', #16222 ) ;
#32892=CARTESIAN_POINT ( 'NONE',  ( -6.123233995736731770E-16, 145.0000000000000568, 27.50000000000000000 ) ) ;
#32901=CIRCLE ( 'NONE', #11348, 3.500000000000003109 ) ;
#32902=CARTESIAN_POINT ( 'NONE',  ( 111.8061974404898962, 19.22934205794938478, 32.50000000000000000 ) ) ;
#32917=ADVANCED_FACE ( 'NONE', ( #33470 ), #14120, .F. ) ;
#32922=LINE ( 'NONE', #13034, #14716 ) ;
#32934=DIRECTION ( 'NONE',  ( -0.000000000000000000, -0.000000000000000000, 1.000000000000000000 ) ) ;
#32936=SHAPE_DEFINITION_REPRESENTATION ( #14547, #6396 ) ;
#32942=CARTESIAN_POINT ( 'NONE',  ( -104.8061974404900241, -19.22934205794863516, 32.50000000000000000 ) ) ;
#32949=EDGE_LOOP ( 'NONE', ( #4889, #32517, #284, #18091 ) ) ;
#32954=ORIENTED_EDGE ( 'NONE', *, *, #14566, .T. ) ;
#32958=DIRECTION ( 'NONE',  ( -1.000000000000000000, 0.000000000000000000, 0.000000000000000000 ) ) ;
#32959=CARTESIAN_POINT ( 'NONE',  ( -79.75042228122002541, 72.37693729083288474, 32.50000000000000000 ) ) ;
#32965=ORIENTED_EDGE ( 'NONE', *, *, #21442, .T. ) ;
#32981=CARTESIAN_POINT ( 'NONE',  ( -107.2742589609544410, 47.50000425637879431, 32.50001250000000397 ) ) ;
#32990=CARTESIAN_POINT ( 'NONE',  ( -94.40806000769299544, 12.15049814296761888, 32.50000000000000000 ) ) ;
#33023=EDGE_CURVE ( 'NONE', #27930, #36161, #14741, .T. ) ;
#33026=DIRECTION ( 'NONE',  ( 0.000000000000000000, 0.000000000000000000, 1.000000000000000000 ) ) ;
#33034=CARTESIAN_POINT ( 'NONE',  ( 37.50000000000000000, -103.4105893997321743, 32.50000000000000000 ) ) ;
#33047=CARTESIAN_POINT ( 'NONE',  ( -105.2710652963492208, -37.58057717672379994, 32.50000000000000711 ) ) ;
#33055=ORIENTED_EDGE ( 'NONE', *, *, #8229, .T. ) ;
#33085=DIRECTION ( 'NONE',  ( 0.000000000000000000, -0.000000000000000000, -1.000000000000000000 ) ) ;
#33089=CIRCLE ( 'NONE', #19923, 95.00000000000001421 ) ;
#33093=PLANE ( 'NONE',  #36524 ) ;
#33119=DIRECTION ( 'NONE',  ( 1.000000000000000000, 0.000000000000000000, 0.000000000000000000 ) ) ;
#33129=AXIS2_PLACEMENT_3D ( 'NONE', #26225, #14417, #535 ) ;
#33130=DIRECTION ( 'NONE',  ( -0.7071067811865439090, 0.7071067811865512365, 0.000000000000000000 ) ) ;
#33151=AXIS2_PLACEMENT_3D ( 'NONE', #19187, #13527, #10737 ) ;
#33155=ORIENTED_EDGE ( 'NONE', *, *, #34019, .F. ) ;
#33170=ORIENTED_EDGE ( 'NONE', *, *, #21867, .T. ) ;
#33171=ORIENTED_EDGE ( 'NONE', *, *, #26597, .F. ) ;
#33173=SURFACE_STYLE_FILL_AREA ( #10139 ) ;
#33187=ORIENTED_EDGE ( 'NONE', *, *, #5384, .T. ) ;
#33194=ORIENTED_EDGE ( 'NONE', *, *, #20191, .F. ) ;
#33198=CIRCLE ( 'NONE', #18324, 30.00000000000000000 ) ;
#33199=CARTESIAN_POINT ( 'NONE',  ( -82.27241335952113843, 47.50000000000096634, 27.50000000000000000 ) ) ;
#33217=EDGE_LOOP ( 'NONE', ( #7370, #7919, #31990, #28830 ) ) ;
#33223=CARTESIAN_POINT ( 'NONE',  ( -101.4252628994512833, -31.43180897937256191, 32.50001250000000397 ) ) ;
#33252=ORIENTED_EDGE ( 'NONE', *, *, #15377, .F. ) ;
#33253=CARTESIAN_POINT ( 'NONE',  ( -110.2237710830543733, -101.7384897088139724, 32.55002500000000509 ) ) ;
#33258=DIRECTION ( 'NONE',  ( -0.000000000000000000, -0.000000000000000000, 1.000000000000000000 ) ) ;
#33260=AXIS2_PLACEMENT_3D ( 'NONE', #28223, #22231, #36665 ) ;
#33266=LINE ( 'NONE', #7584, #20526 ) ;
#33301=ADVANCED_FACE ( 'NONE', ( #5295 ), #10529, .F. ) ;
#33320=AXIS2_PLACEMENT_3D ( 'NONE', #24975, #22329, #17067 ) ;
#33322=LINE ( 'NONE', #16267, #14224 ) ;
#33327=CARTESIAN_POINT ( 'NONE',  ( -107.2742589609544410, 47.50000425637879431, 32.50001250000000397 ) ) ;
#33347=LINE ( 'NONE', #4673, #18219 ) ;
#33349=DIRECTION ( 'NONE',  ( -0.000000000000000000, -0.000000000000000000, 1.000000000000000000 ) ) ;
#33362=DIRECTION ( 'NONE',  ( 1.000000000000000000, 0.000000000000000000, 0.000000000000000000 ) ) ;
#33370=CARTESIAN_POINT ( 'NONE',  ( -104.5390599191612182, -58.87763622169656941, 32.50000000000000000 ) ) ;
#33378=SURFACE_STYLE_USAGE ( .BOTH. , #7881 ) ;
#33384=CIRCLE ( 'NONE', #1660, 30.00000000000000000 ) ;
#33391=VERTEX_POINT ( 'NONE', #5091 ) ;
#33425=CARTESIAN_POINT ( 'NONE',  ( 37.50000000000000000, -103.4105893997321743, 32.50000000000000000 ) ) ;
#33426=CARTESIAN_POINT ( 'NONE',  ( 149.8799519615616020, -6.000000000000508038, 27.50000000000000000 ) ) ;
#33427=EDGE_CURVE ( 'NONE', #40, #7276, #27963, .T. ) ;
#33437=ORIENTED_EDGE ( 'NONE', *, *, #34206, .T. ) ;
#33444=ORIENTED_EDGE ( 'NONE', *, *, #23414, .F. ) ;
#33449=DIRECTION ( 'NONE',  ( -0.000000000000000000, -0.000000000000000000, 1.000000000000000000 ) ) ;
#33463=CARTESIAN_POINT ( 'NONE',  ( -16.42335909229131374, 114.0197456316801237, 27.49998799999999477 ) ) ;
#33467=ORIENTED_EDGE ( 'NONE', *, *, #29664, .T. ) ;
#33470=FACE_OUTER_BOUND ( 'NONE', #18674, .T. ) ;
#33472=VECTOR ( 'NONE', #11455, 1000.000000000000000 ) ;
#33476=EDGE_LOOP ( 'NONE', ( #3306, #37052 ) ) ;
#33496=CARTESIAN_POINT ( 'NONE',  ( -34.00000000000000000, -103.4105893997321743, 32.50000000000000000 ) ) ;
#33499=LINE ( 'NONE', #16416, #34461 ) ;
#33500=DIRECTION ( 'NONE',  ( 1.000000000000000000, 1.422473250300981817E-14, 0.000000000000000000 ) ) ;
#33512=VECTOR ( 'NONE', #35646, 1000.000000000000000 ) ;
#33517=CIRCLE ( 'NONE', #15518, 3.500000000000003109 ) ;
#33574=DIRECTION ( 'NONE',  ( 0.000000000000000000, 0.000000000000000000, 1.000000000000000000 ) ) ;
#33581=DIRECTION ( 'NONE',  ( 0.000000000000000000, 0.000000000000000000, 1.000000000000000000 ) ) ;
#33593=EDGE_CURVE ( 'NONE', #24047, #20316, #11613, .T. ) ;
#33600=DIRECTION ( 'NONE',  ( -0.000000000000000000, -0.000000000000000000, 1.000000000000000000 ) ) ;
#33604=ADVANCED_FACE ( 'NONE', ( #27168 ), #24378, .F. ) ;
#33641=CARTESIAN_POINT ( 'NONE',  ( -34.00000000000000000, 103.4105893997321743, 32.50000000000000000 ) ) ;
#33644=CARTESIAN_POINT ( 'NONE',  ( 2.545083245400402649, 119.9999999808429294, 27.49998800000000188 ) ) ;
#33678=CARTESIAN_POINT ( 'NONE',  ( 67.30619744049005249, 84.18124734178236679, 32.50000000000000000 ) ) ;
#33683=AXIS2_PLACEMENT_3D ( 'NONE', #25530, #25184, #7916 ) ;
#33690=ORIENTED_EDGE ( 'NONE', *, *, #6435, .T. ) ;
#33700=DIRECTION ( 'NONE',  ( -0.000000000000000000, -0.000000000000000000, 1.000000000000000000 ) ) ;
#33706=EDGE_CURVE ( 'NONE', #13025, #17798, #31541, .T. ) ;
#33727=ORIENTED_EDGE ( 'NONE', *, *, #8737, .F. ) ;
#33745=( NAMED_UNIT ( * ) SI_UNIT ( $, .STERADIAN. ) SOLID_ANGLE_UNIT ( ) );
#33750=ORIENTED_EDGE ( 'NONE', *, *, #29584, .F. ) ;
#33763=ORIENTED_EDGE ( 'NONE', *, *, #14456, .F. ) ;
#33765=EDGE_CURVE ( 'NONE', #23824, #18795, #11226, .T. ) ;
#33766=ORIENTED_EDGE ( 'NONE', *, *, #12311, .F. ) ;
#33798=EDGE_CURVE ( 'NONE', #28579, #10948, #11208, .T. ) ;
#33826=ORIENTED_EDGE ( 'NONE', *, *, #2006, .T. ) ;
#33841=ORIENTED_EDGE ( 'NONE', *, *, #33865, .T. ) ;
#33846=DIRECTION ( 'NONE',  ( 0.000000000000000000, 0.000000000000000000, 1.000000000000000000 ) ) ;
#33855=VERTEX_POINT ( 'NONE', #16138 ) ;
#33862=CIRCLE ( 'NONE', #35063, 25.00000000000000000 ) ;
#33864=COLOUR_RGB ( '', 0.66274510, 0.83137255, 0.94901961) ;
#33865=EDGE_CURVE ( 'NONE', #20872, #22736, #10862, .T. ) ;
#33868=DIRECTION ( 'NONE',  ( -0.000000000000000000, -0.000000000000000000, 1.000000000000000000 ) ) ;
#33879=VERTEX_POINT ( 'NONE', #16309 ) ;
#33881=ORIENTED_EDGE ( 'NONE', *, *, #13231, .F. ) ;
#33895=LINE ( 'NONE', #5570, #35300 ) ;
#33902=ORIENTED_EDGE ( 'NONE', *, *, #8726, .F. ) ;
#33907=EDGE_CURVE ( 'NONE', #13265, #36317, #33384, .T. ) ;
#33916=CIRCLE ( 'NONE', #32697, 30.00000000000000000 ) ;
#33922=CARTESIAN_POINT ( 'NONE',  ( 88.66502283662251216, -71.67713940050370525, 32.50000000000000000 ) ) ;
#33923=CARTESIAN_POINT ( 'NONE',  ( -97.64058335231293029, -67.22370022648394183, 32.49999999999999289 ) ) ;
#33953=ORIENTED_EDGE ( 'NONE', *, *, #4764, .T. ) ;
#33991=EDGE_CURVE ( 'NONE', #31244, #17078, #5595, .T. ) ;
#33993=EDGE_CURVE ( 'NONE', #7521, #17956, #6326, .T. ) ;
#33996=ADVANCED_FACE ( 'NONE', ( #22855 ), #34123, .T. ) ;
#34019=EDGE_CURVE ( 'NONE', #22880, #18795, #14223, .T. ) ;
#34023=AXIS2_PLACEMENT_3D ( 'NONE', #35873, #991, #9792 ) ;
#34035=DIRECTION ( 'NONE',  ( -0.000000000000000000, -0.000000000000000000, -1.000000000000000000 ) ) ;
#34042=CARTESIAN_POINT ( 'NONE',  ( 14.38872371163433428, -115.5691697732052177, 32.49999999999999289 ) ) ;
#34046=EDGE_LOOP ( 'NONE', ( #22797, #4141, #9754, #29852 ) ) ;
#34059=CARTESIAN_POINT ( 'NONE',  ( 72.72667006429115588, 101.6652913307178636, 32.50002500000000083 ) ) ;
#34061=CARTESIAN_POINT ( 'NONE',  ( 23.49187040204899546, -103.5527524078059400, 32.50001250000000397 ) ) ;
#34105=VECTOR ( 'NONE', #30788, 1000.000000000000000 ) ;
#34107=DIRECTION ( 'NONE',  ( 0.000000000000000000, 0.000000000000000000, 1.000000000000000000 ) ) ;
#34110=CIRCLE ( 'NONE', #31096, 3.499999999999996003 ) ;
#34121=CARTESIAN_POINT ( 'NONE',  ( 77.93337651276290501, -72.12094976675109592, 32.50001250000000397 ) ) ;
#34123=CYLINDRICAL_SURFACE ( 'NONE', #26787, 150.0000000000000284 ) ;
#34124=CARTESIAN_POINT ( 'NONE',  ( 108.3061974404898820, 19.22934205794938478, 32.50000000000000000 ) ) ;
#34140=CIRCLE ( 'NONE', #5393, 6.000000000000005329 ) ;
#34142=ADVANCED_FACE ( 'NONE', ( #24665 ), #1589, .F. ) ;
#34150=AXIS2_PLACEMENT_3D ( 'NONE', #19709, #30943, #36763 ) ;
#34180=CARTESIAN_POINT ( 'NONE',  ( 0.000000000000000000, 0.000000000000000000, 32.50000000000000000 ) ) ;
#34181=ADVANCED_FACE ( 'NONE', ( #27469 ), #27087, .F. ) ;
#34205=CARTESIAN_POINT ( 'NONE',  ( -67.30619744049063513, -84.18124734178186941, 32.50000000000000000 ) ) ;
#34206=EDGE_CURVE ( 'NONE', #10748, #3694, #29100, .T. ) ;
#34209=CARTESIAN_POINT ( 'NONE',  ( 16.42335937861835049, 114.0197453844396591, 27.49998800000000898 ) ) ;
#34210=EDGE_CURVE ( 'NONE', #32620, #9158, #21947, .T. ) ;
#34227=CARTESIAN_POINT ( 'NONE',  ( 22.49971464476085359, -105.9191578779291802, 32.49999999999999289 ) ) ;
#34232=CARTESIAN_POINT ( 'NONE',  ( -124.4080600076929954, 12.15049814296761888, 32.50000000000000000 ) ) ;
#34238=DIRECTION ( 'NONE',  ( 0.000000000000000000, -0.000000000000000000, -1.000000000000000000 ) ) ;
#34253=DIRECTION ( 'NONE',  ( 1.000000000000000000, 0.000000000000000000, 0.000000000000000000 ) ) ;
#34255=EDGE_LOOP ( 'NONE', ( #34260, #1657 ) ) ;
#34260=ORIENTED_EDGE ( 'NONE', *, *, #26982, .F. ) ;
#34262=CARTESIAN_POINT ( 'NONE',  ( -104.8061974404896262, 19.22934205795090534, 32.50000000000000000 ) ) ;
#34265=ORIENTED_EDGE ( 'NONE', *, *, #1403, .F. ) ;
#34303=CIRCLE ( 'NONE', #7350, 150.0000000000000284 ) ;
#34313=EDGE_LOOP ( 'NONE', ( #12859, #1398, #29172, #17431 ) ) ;
#34390=DIRECTION ( 'NONE',  ( 1.000000000000000000, 0.000000000000000000, 0.000000000000000000 ) ) ;
#34414=DIRECTION ( 'NONE',  ( -0.000000000000000000, -0.000000000000000000, -1.000000000000000000 ) ) ;
#34423=DIRECTION ( 'NONE',  ( 1.000000000000000000, 0.000000000000000000, 0.000000000000000000 ) ) ;
#34461=VECTOR ( 'NONE', #10965, 1000.000000000000000 ) ;
#34462=CIRCLE ( 'NONE', #36865, 3.500000000000003109 ) ;
#34470=FACE_OUTER_BOUND ( 'NONE', #10253, .T. ) ;
#34473=B_SPLINE_CURVE_WITH_KNOTS ( 'NONE', 3,
 ( #8424, #10860, #36732, #27723, #5043, #25678, #10482, #22297, #16857, #30908, #22468, #8239, #33923, #28278, #2598, #21926, #14026, #25474, #19851, #33370, #36913, #11224, #22673, #31272, #5594, #17965, #11569, #31987 ),
 .UNSPECIFIED., .F., .F.,
 ( 4, 2, 1, 2, 2, 1, 1, 2, 2, 1, 2, 2, 1, 1, 2, 2, 4 ),
 ( 0.05563282717593193150, 0.06430909872693714446, 0.07298537027794235743, 0.09033791337995278337, 0.1250429995839733577, 0.1597480857879939320, 0.1771006288900040526, 0.1857769004410091129, 0.1944531719920141732, 0.2291582581960339982, 0.2465108012980439245, 0.2551870728490489015, 0.2638633444000538786, 0.2985684306040737868, 0.3072447021550788193, 0.3159209737060837964, 0.3332735168080938615 ),
 .UNSPECIFIED. ) ;
#34489=ORIENTED_EDGE ( 'NONE', *, *, #35582, .T. ) ;
#34516=DIRECTION ( 'NONE',  ( 0.000000000000000000, 0.000000000000000000, 1.000000000000000000 ) ) ;
#34519=VERTEX_POINT ( 'NONE', #16182 ) ;
#34525=LINE ( 'NONE', #14830, #33472 ) ;
#34533=VECTOR ( 'NONE', #36605, 1000.000000000000000 ) ;
#34534=DIRECTION ( 'NONE',  ( 0.000000000000000000, -0.000000000000000000, -1.000000000000000000 ) ) ;
#34547=AXIS2_PLACEMENT_3D ( 'NONE', #33199, #35308, #15600 ) ;
#34557=CARTESIAN_POINT ( 'NONE',  ( 98.21839120950853896, -66.76535579868571801, 32.50000000000000000 ) ) ;
#34570=CARTESIAN_POINT ( 'NONE',  ( -111.8061974404896262, 19.22934205795090534, 32.50000000000000000 ) ) ;
#34589=CARTESIAN_POINT ( 'NONE',  ( -12.20857224668173480, -116.8572664861451642, 32.50000000000000711 ) ) ;
#34598=CARTESIAN_POINT ( 'NONE',  ( -110.2237710830522559, 101.7384897088162745, 27.50000000000000000 ) ) ;
#34613=CIRCLE ( 'NONE', #17259, 95.00000000000001421 ) ;
#34616=DIRECTION ( 'NONE',  ( 1.000000000000000000, 0.000000000000000000, 0.000000000000000000 ) ) ;
#34631=AXIS2_PLACEMENT_3D ( 'NONE', #14908, #5927, #28781 ) ;
#34641=EDGE_CURVE ( 'NONE', #2865, #5973, #19910, .T. ) ;
#34665=LINE ( 'NONE', #32557, #30902 ) ;
#34666=EDGE_CURVE ( 'NONE', #1946, #13968, #6739, .T. ) ;
#34686=AXIS2_PLACEMENT_3D ( 'NONE', #30539, #13275, #21905 ) ;
#34690=DIRECTION ( 'NONE',  ( -0.000000000000000000, -0.000000000000000000, 1.000000000000000000 ) ) ;
#34705=DIRECTION ( 'NONE',  ( 0.000000000000000000, 0.000000000000000000, 1.000000000000000000 ) ) ;
#34706=DIRECTION ( 'NONE',  ( -0.000000000000000000, -0.000000000000000000, 1.000000000000000000 ) ) ;
#34712=EDGE_CURVE ( 'NONE', #3789, #5373, #32483, .T. ) ;
#34727=CARTESIAN_POINT ( 'NONE',  ( 95.00000000000001421, 0.000000000000000000, 32.50000000000000000 ) ) ;
#34736=EDGE_CURVE ( 'NONE', #17798, #13025, #144, .T. ) ;
#34743=CIRCLE ( 'NONE', #3020, 6.000000000000005329 ) ;
#34751=DIRECTION ( 'NONE',  ( 0.000000000000000000, -0.000000000000000000, -1.000000000000000000 ) ) ;
#34754=DIRECTION ( 'NONE',  ( 0.000000000000000000, 0.000000000000000000, 1.000000000000000000 ) ) ;
#34762=AXIS2_PLACEMENT_3D ( 'NONE', #32418, #6920, #6732 ) ;
#34786=DIRECTION ( 'NONE',  ( 1.000000000000000000, 0.000000000000000000, 0.000000000000000000 ) ) ;
#34792=ORIENTED_EDGE ( 'NONE', *, *, #4659, .F. ) ;
#34807=CIRCLE ( 'NONE', #16843, 6.000000000000005329 ) ;
#34816=ORIENTED_EDGE ( 'NONE', *, *, #26345, .T. ) ;
#34821=CARTESIAN_POINT ( 'NONE',  ( -6.000000000000000000, 0.000000000000000000, 27.50000000000000000 ) ) ;
#34876=CARTESIAN_POINT ( 'NONE',  ( 23.49188653442568864, 103.5527583403323035, 27.49999400000000094 ) ) ;
#34877=CARTESIAN_POINT ( 'NONE',  ( 106.2299706463093827, 40.32678131133052801, 32.50000000000000000 ) ) ;
#34914=DIRECTION ( 'NONE',  ( 1.000000000000000000, 0.000000000000000000, 0.000000000000000000 ) ) ;
#34923=CARTESIAN_POINT ( 'NONE',  ( -6.000000000000000000, 145.0000000000000568, 32.55002500000000509 ) ) ;
#34936=CARTESIAN_POINT ( 'NONE',  ( 96.53048327204888324, -102.5304832720499633, 32.55002500000000509 ) ) ;
#34944=FACE_OUTER_BOUND ( 'NONE', #6513, .T. ) ;
#34950=DIRECTION ( 'NONE',  ( -0.000000000000000000, -0.000000000000000000, 1.000000000000000000 ) ) ;
#34953=EDGE_CURVE ( 'NONE', #8678, #8665, #21380, .T. ) ;
#34969=VECTOR ( 'NONE', #9853, 1000.000000000000000 ) ;
#34971=VECTOR ( 'NONE', #25176, 1000.000000000000000 ) ;
#34976=DIRECTION ( 'NONE',  ( 1.000000000000000000, 0.000000000000000000, 0.000000000000000000 ) ) ;
#34994=DIRECTION ( 'NONE',  ( 0.000000000000000000, -0.000000000000000000, -1.000000000000000000 ) ) ;
#34995=AXIS2_PLACEMENT_3D ( 'NONE', #32032, #3381, #35628 ) ;
#35001=DIRECTION ( 'NONE',  ( 0.000000000000000000, 0.000000000000000000, 1.000000000000000000 ) ) ;
#35012=ORIENTED_EDGE ( 'NONE', *, *, #36316, .T. ) ;
#35021=DIRECTION ( 'NONE',  ( -0.000000000000000000, -0.000000000000000000, 1.000000000000000000 ) ) ;
#35034=ORIENTED_EDGE ( 'NONE', *, *, #36344, .F. ) ;
#35039=AXIS2_PLACEMENT_3D ( 'NONE', #20380, #303, #31965 ) ;
#35059=CARTESIAN_POINT ( 'NONE',  ( 79.20400555976016221, 72.31907731944103546, 32.50000000000000000 ) ) ;
#35062=ORIENTED_EDGE ( 'NONE', *, *, #23389, .F. ) ;
#35063=AXIS2_PLACEMENT_3D ( 'NONE', #16275, #30867, #4657 ) ;
#35080=FACE_BOUND ( 'NONE', #32185, .T. ) ;
#35089=VECTOR ( 'NONE', #1963, 1000.000000000000000 ) ;
#35097=ADVANCED_FACE ( 'NONE', ( #24752 ), #2606, .F. ) ;
#35101=CARTESIAN_POINT ( 'NONE',  ( -106.6136999110908476, 41.75147322074028722, 32.50000000000000000 ) ) ;
#35109=LINE ( 'NONE', #29457, #20830 ) ;
#35112=VERTEX_POINT ( 'NONE', #22480 ) ;
#35116=AXIS2_PLACEMENT_3D ( 'NONE', #15005, #12347, #17807 ) ;
#35141=LINE ( 'NONE', #32312, #6585 ) ;
#35173=CYLINDRICAL_SURFACE ( 'NONE', #24385, 150.0000000000000284 ) ;
#35188=AXIS2_PLACEMENT_3D ( 'NONE', #26157, #22979, #37055 ) ;
#35190=DIRECTION ( 'NONE',  ( -0.000000000000000000, -0.000000000000000000, 1.000000000000000000 ) ) ;
#35198=CARTESIAN_POINT ( 'NONE',  ( -77.93337651276257816, 72.12094976675054170, 32.50001250000000397 ) ) ;
#35214=CARTESIAN_POINT ( 'NONE',  ( -6.000000000000000000, 149.8799519615616305, 32.50000000000000000 ) ) ;
#35215=CARTESIAN_POINT ( 'NONE',  ( 6.000000000000000000, -149.8799519615616305, 32.50000000000000000 ) ) ;
#35219=EDGE_CURVE ( 'NONE', #17144, #19856, #23228, .T. ) ;
#35222=CARTESIAN_POINT ( 'NONE',  ( 77.93343913441647430, -72.12058696850856165, 27.50000000000000000 ) ) ;
#35223=CARTESIAN_POINT ( 'NONE',  ( -23.49154088336464952, -103.5526315789473699, 32.50002500000000083 ) ) ;
#35229=AXIS2_PLACEMENT_3D ( 'NONE', #15668, #4411, #12257 ) ;
#35246=CARTESIAN_POINT ( 'NONE',  ( 4.242640687119251908, -4.242640687119325626, 32.50000000000000000 ) ) ;
#35247=EDGE_LOOP ( 'NONE', ( #7920, #5424, #26650, #10105 ) ) ;
#35248=AXIS2_PLACEMENT_3D ( 'NONE', #16462, #30887, #27893 ) ;
#35253=CARTESIAN_POINT ( 'NONE',  ( 145.0000000000000568, -5.056524707326808249E-13, 27.50000000000000000 ) ) ;
#35268=CARTESIAN_POINT ( 'NONE',  ( 104.0325470118518751, 35.06873771483363100, 32.49999999999999289 ) ) ;
#35270=AXIS2_PLACEMENT_3D ( 'NONE', #8470, #6195, #16906 ) ;
#35290=FACE_BOUND ( 'NONE', #34255, .T. ) ;
#35291=DIRECTION ( 'NONE',  ( -0.000000000000000000, -0.000000000000000000, -1.000000000000000000 ) ) ;
#35295=DIRECTION ( 'NONE',  ( 1.000000000000000000, 0.000000000000000000, 0.000000000000000000 ) ) ;
#35300=VECTOR ( 'NONE', #23196, 1000.000000000000000 ) ;
#35306=EDGE_CURVE ( 'NONE', #10807, #11432, #12143, .T. ) ;
#35308=DIRECTION ( 'NONE',  ( 0.000000000000000000, 0.000000000000000000, 1.000000000000000000 ) ) ;
#35309=CIRCLE ( 'NONE', #26915, 3.500000000000003109 ) ;
#35326=VECTOR ( 'NONE', #13042, 999.9999999999998863 ) ;
#35334=CIRCLE ( 'NONE', #3596, 6.000000000000005329 ) ;
#35340=CARTESIAN_POINT ( 'NONE',  ( 9.904614206369521057, -117.9630559560052632, 32.49999999999999289 ) ) ;
#35355=VECTOR ( 'NONE', #18102, 1000.000000000000000 ) ;
#35382=ORIENTED_EDGE ( 'NONE', *, *, #20366, .F. ) ;
#35387=DIRECTION ( 'NONE',  ( -0.000000000000000000, -0.000000000000000000, -1.000000000000000000 ) ) ;
#35406=DIRECTION ( 'NONE',  ( 1.000000000000000000, 0.000000000000000000, 0.000000000000000000 ) ) ;
#35430=DIRECTION ( 'NONE',  ( 0.7071067811865536790, 0.7071067811865414665, 0.000000000000000000 ) ) ;
#35436=ADVANCED_FACE ( 'NONE', ( #3889 ), #26578, .T. ) ;
#35458=DIRECTION ( 'NONE',  ( -0.000000000000000000, -0.000000000000000000, 1.000000000000000000 ) ) ;
#35502=CYLINDRICAL_SURFACE ( 'NONE', #34023, 95.00000000000001421 ) ;
#35512=VERTEX_POINT ( 'NONE', #29564 ) ;
#35519=FACE_OUTER_BOUND ( 'NONE', #10118, .T. ) ;
#35528=LINE ( 'NONE', #18082, #13612 ) ;
#35545=VECTOR ( 'NONE', #14319, 1000.000000000000000 ) ;
#35557=FACE_BOUND ( 'NONE', #31259, .T. ) ;
#35564=CARTESIAN_POINT ( 'NONE',  ( 94.55012560584681580, 9.234378588654081454, 27.50000000000000000 ) ) ;
#35575=FACE_OUTER_BOUND ( 'NONE', #20015, .T. ) ;
#35582=EDGE_CURVE ( 'NONE', #23728, #32620, #33862, .T. ) ;
#35594=EDGE_CURVE ( 'NONE', #35608, #17798, #19446, .T. ) ;
#35601=CARTESIAN_POINT ( 'NONE',  ( -145.0000000000001137, -5.999999999998481215, 32.55002500000000509 ) ) ;
#35608=VERTEX_POINT ( 'NONE', #2570 ) ;
#35609=CARTESIAN_POINT ( 'NONE',  ( -23.49154088336464952, 103.5526315789473699, 32.50000000000000000 ) ) ;
#35619=CARTESIAN_POINT ( 'NONE',  ( -37.50000000000000000, -103.4105893997321743, 27.50000000000000000 ) ) ;
#35628=DIRECTION ( 'NONE',  ( 1.000000000000000000, 0.000000000000000000, 0.000000000000000000 ) ) ;
#35642=CARTESIAN_POINT ( 'NONE',  ( -124.4080600076929954, 12.15049814296761888, 32.50002500000000083 ) ) ;
#35646=DIRECTION ( 'NONE',  ( -0.000000000000000000, -0.000000000000000000, 1.000000000000000000 ) ) ;
#35675=DIRECTION ( 'NONE',  ( 1.000000000000000000, 0.000000000000000000, 0.000000000000000000 ) ) ;
#35680=VERTEX_POINT ( 'NONE', #34262 ) ;
#35684=VECTOR ( 'NONE', #34534, 1000.000000000000000 ) ;
#35686=CARTESIAN_POINT ( 'NONE',  ( 6.000000000000000000, -145.0000000000000568, 32.50000000000000000 ) ) ;
#35701=AXIS2_PLACEMENT_3D ( 'NONE', #2927, #2720, #22973 ) ;
#35710=DIRECTION ( 'NONE',  ( 1.000000000000000000, 0.000000000000000000, 0.000000000000000000 ) ) ;
#35711=DIRECTION ( 'NONE',  ( 0.000000000000000000, 0.000000000000000000, 1.000000000000000000 ) ) ;
#35726=VERTEX_POINT ( 'NONE', #491 ) ;
#35732=AXIS2_PLACEMENT_3D ( 'NONE', #32892, #7212, #30063 ) ;
#35736=DIRECTION ( 'NONE',  ( -0.000000000000000000, -0.000000000000000000, -1.000000000000000000 ) ) ;
#35738=DIRECTION ( 'NONE',  ( -1.000000000000000000, 0.000000000000000000, 0.000000000000000000 ) ) ;
#35773=DIRECTION ( 'NONE',  ( 1.000000000000000000, 0.000000000000000000, 0.000000000000000000 ) ) ;
#35778=VERTEX_POINT ( 'NONE', #14185 ) ;
#35783=EDGE_CURVE ( 'NONE', #27651, #20315, #17192, .T. ) ;
#35791=ORIENTED_EDGE ( 'NONE', *, *, #29895, .T. ) ;
#35802=FACE_OUTER_BOUND ( 'NONE', #19554, .T. ) ;
#35808=EDGE_CURVE ( 'NONE', #10982, #17563, #32922, .T. ) ;
#35830=ORIENTED_EDGE ( 'NONE', *, *, #26497, .T. ) ;
#35841=ORIENTED_EDGE ( 'NONE', *, *, #24800, .T. ) ;
#35843=CARTESIAN_POINT ( 'NONE',  ( 0.000000000000000000, 0.000000000000000000, 27.50000000000000000 ) ) ;
#35848=DIRECTION ( 'NONE',  ( -0.7071067811865487940, -0.7071067811865463515, 0.000000000000000000 ) ) ;
#35849=ORIENTED_EDGE ( 'NONE', *, *, #35594, .T. ) ;
#35850=ORIENTED_EDGE ( 'NONE', *, *, #26982, .T. ) ;
#35851=CIRCLE ( 'NONE', #31129, 3.499999999999996003 ) ;
#35854=FACE_OUTER_BOUND ( 'NONE', #34046, .T. ) ;
#35873=CARTESIAN_POINT ( 'NONE',  ( 0.000000000000000000, 0.000000000000000000, 27.50000000000000000 ) ) ;
#35891=VECTOR ( 'NONE', #26384, 1000.000000000000000 ) ;
#35902=AXIS2_PLACEMENT_3D ( 'NONE', #2351, #16402, #4962 ) ;
#35923=EDGE_CURVE ( 'NONE', #13732, #13259, #12264, .T. ) ;
#35925=FACE_OUTER_BOUND ( 'NONE', #14501, .T. ) ;
#35933=EDGE_CURVE ( 'NONE', #35680, #30153, #8139, .T. ) ;
#35937=CIRCLE ( 'NONE', #35270, 3.500000000000003109 ) ;
#35944=CARTESIAN_POINT ( 'NONE',  ( -70.80619744049063513, -84.18124734178186941, 32.50000000000000000 ) ) ;
#35972=CARTESIAN_POINT ( 'NONE',  ( -90.52737013603423577, 71.16947008734744884, 32.50000000000000000 ) ) ;
#35973=ORIENTED_EDGE ( 'NONE', *, *, #24447, .F. ) ;
#36022=EDGE_CURVE ( 'NONE', #5071, #30149, #7412, .T. ) ;
#36031=CARTESIAN_POINT ( 'NONE',  ( 124.4080600076930665, -12.15049814296675201, 32.50000000000000000 ) ) ;
#36078=AXIS2_PLACEMENT_3D ( 'NONE', #23106, #3229, #17481 ) ;
#36104=ADVANCED_FACE ( 'NONE', ( #29440, #6586, #18018, #17828, #23636, #20446, #26629, #35080, #18188, #6200, #25899, #35290, #28880, #17627 ), #14835, .T. ) ;
#36106=FACE_BOUND ( 'NONE', #17687, .T. ) ;
#36115=CYLINDRICAL_SURFACE ( 'NONE', #22434, 30.00000000000000000 ) ;
#36131=CARTESIAN_POINT ( 'NONE',  ( 106.7731239591682026, -98.28784258493070070, 32.50000000000000000 ) ) ;
#36139=CARTESIAN_POINT ( 'NONE',  ( -104.5389608366994167, 58.87775083094626183, 32.49999999999999289 ) ) ;
#36154=VERTEX_POINT ( 'NONE', #34727 ) ;
#36161=VERTEX_POINT ( 'NONE', #6755 ) ;
#36198=LINE ( 'NONE', #10320, #33512 ) ;
#36217=CARTESIAN_POINT ( 'NONE',  ( -106.7731239591695669, -98.28784258492920856, 32.55002500000000509 ) ) ;
#36222=DIRECTION ( 'NONE',  ( 1.000000000000000000, 0.000000000000000000, 0.000000000000000000 ) ) ;
#36224=AXIS2_PLACEMENT_3D ( 'NONE', #29973, #12530, #9905 ) ;
#36226=AXIS2_PLACEMENT_3D ( 'NONE', #5611, #34690, #11777 ) ;
#36246=FACE_OUTER_BOUND ( 'NONE', #22698, .T. ) ;
#36253=EDGE_CURVE ( 'NONE', #34519, #13060, #33916, .T. ) ;
#36259=LINE ( 'NONE', #30243, #11723 ) ;
#36274=AXIS2_PLACEMENT_3D ( 'NONE', #34923, #9217, #20649 ) ;
#36284=DIRECTION ( 'NONE',  ( -3.554796214472773777E-16, -1.000000000000000000, 0.000000000000000000 ) ) ;
#36298=CIRCLE ( 'NONE', #27284, 25.00000000000000000 ) ;
#36310=LINE ( 'NONE', #33678, #31607 ) ;
#36316=EDGE_CURVE ( 'NONE', #29025, #13349, #34665, .T. ) ;
#36317=VERTEX_POINT ( 'NONE', #35222 ) ;
#36331=CARTESIAN_POINT ( 'NONE',  ( -98.00091034470435147, 66.93791212686957692, 32.50000000000000711 ) ) ;
#36344=EDGE_CURVE ( 'NONE', #27555, #1358, #29693, .T. ) ;
#36364=EDGE_LOOP ( 'NONE', ( #35841, #28172, #17043, #14996 ) ) ;
#36374=CARTESIAN_POINT ( 'NONE',  ( 40.99999999999999289, -103.4105893997321743, 27.50000000000000000 ) ) ;
#36387=VECTOR ( 'NONE', #3536, 1000.000000000000000 ) ;
#36394=ORIENTED_EDGE ( 'NONE', *, *, #11654, .F. ) ;
#36396=DIRECTION ( 'NONE',  ( 1.000000000000000000, 0.000000000000000000, 0.000000000000000000 ) ) ;
#36484=CARTESIAN_POINT ( 'NONE',  ( 110.2237710830529664, -101.7384897088154929, 32.50000000000000000 ) ) ;
#36485=VERTEX_POINT ( 'NONE', #27506 ) ;
#36494=AXIS2_PLACEMENT_3D ( 'NONE', #436, #6442, #5902 ) ;
#36508=FACE_OUTER_BOUND ( 'NONE', #27998, .T. ) ;
#36513=AXIS2_PLACEMENT_3D ( 'NONE', #7983, #7814, #10618 ) ;
#36524=AXIS2_PLACEMENT_3D ( 'NONE', #30094, #16406, #18854 ) ;
#36525=ORIENTED_EDGE ( 'NONE', *, *, #14456, .T. ) ;
#36530=ORIENTED_EDGE ( 'NONE', *, *, #17633, .F. ) ;
#36586=ORIENTED_EDGE ( 'NONE', *, *, #6260, .T. ) ;
#36592=CARTESIAN_POINT ( 'NONE',  ( 6.000000000000000000, -145.0000000000000568, 27.50000000000000000 ) ) ;
#36605=DIRECTION ( 'NONE',  ( 0.7071067811865435759, -0.7071067811865514585, 0.000000000000000000 ) ) ;
#36608=ADVANCED_FACE ( 'NONE', ( #25626 ), #8379, .F. ) ;
#36617=ADVANCED_FACE ( 'NONE', ( #19625 ), #16429, .F. ) ;
#36644=DIRECTION ( 'NONE',  ( -1.000000000000000000, 0.000000000000000000, 0.000000000000000000 ) ) ;
#36650=ORIENTED_EDGE ( 'NONE', *, *, #14639, .F. ) ;
#36665=DIRECTION ( 'NONE',  ( 1.000000000000000000, 1.792547591842699744E-15, 0.000000000000000000 ) ) ;
#36671=DIRECTION ( 'NONE',  ( 1.000000000000000000, 0.000000000000000000, 0.000000000000000000 ) ) ;
#36672=ADVANCED_FACE ( 'NONE', ( #19430 ), #28407, .T. ) ;
#36674=DIRECTION ( 'NONE',  ( -1.000000000000000000, 0.000000000000000000, 0.000000000000000000 ) ) ;
#36687=ADVANCED_FACE ( 'NONE', ( #25255 ), #22419, .F. ) ;
#36704=ADVANCED_FACE ( 'NONE', ( #14168 ), #4422, .F. ) ;
#36719=CARTESIAN_POINT ( 'NONE',  ( 101.4249800177813086, -31.43204461043964315, 27.50000000000000000 ) ) ;
#36729=EDGE_CURVE ( 'NONE', #12147, #8890, #29722, .T. ) ;
#36732=CARTESIAN_POINT ( 'NONE',  ( -78.83864671358962539, -72.26719042872781529, 32.49999999999999289 ) ) ;
#36733=CARTESIAN_POINT ( 'NONE',  ( 94.40806000769313755, 12.15049814296589226, 32.50002500000000083 ) ) ;
#36734=CARTESIAN_POINT ( 'NONE',  ( 0.000000000000000000, 0.000000000000000000, 27.50000000000000000 ) ) ;
#36744=ORIENTED_EDGE ( 'NONE', *, *, #24988, .T. ) ;
#36748=CIRCLE ( 'NONE', #20557, 3.499999999999996003 ) ;
#36761=DIRECTION ( 'NONE',  ( -1.000000000000000000, 3.491481338843133750E-15, 0.000000000000000000 ) ) ;
#36763=DIRECTION ( 'NONE',  ( 1.000000000000000000, 0.000000000000000000, 0.000000000000000000 ) ) ;
#36765=DIRECTION ( 'NONE',  ( 1.000000000000000000, 0.000000000000000000, 0.000000000000000000 ) ) ;
#36781=CARTESIAN_POINT ( 'NONE',  ( -106.2329258812508641, -40.32806679316945520, 32.50000000000000000 ) ) ;
#36790=EDGE_CURVE ( 'NONE', #27821, #29329, #5812, .T. ) ;
#36791=DIRECTION ( 'NONE',  ( 1.000000000000000000, 9.251858538542971828E-16, 0.000000000000000000 ) ) ;
#36798=LINE ( 'NONE', #5121, #15955 ) ;
#36803=EDGE_LOOP ( 'NONE', ( #28334, #24234, #9377, #29537 ) ) ;
#36813=CIRCLE ( 'NONE', #28998, 30.00000000000000000 ) ;
#36835=ORIENTED_EDGE ( 'NONE', *, *, #35219, .T. ) ;
#36863=B_SPLINE_CURVE_WITH_KNOTS ( 'NONE', 3,
 ( #2481, #1918, #25348, #30774, #36781, #21617, #33047, #13175, #1739, #5100, #27972, #33223 ),
 .UNSPECIFIED., .F., .F.,
 ( 4, 1, 2, 2, 1, 2, 4 ),
 ( 0.3332735168080938615, 0.3610471732601487904, 0.3749340014861762826, 0.3888208297122037749, 0.4165944861642589259, 0.4304813143902864181, 0.4443681426163139103 ),
 .UNSPECIFIED. ) ;
#36865=AXIS2_PLACEMENT_3D ( 'NONE', #17292, #26078, #31329 ) ;
#36883=AXIS2_PLACEMENT_3D ( 'NONE', #35642, #18395, #12569 ) ;
#36886=CARTESIAN_POINT ( 'NONE',  ( 0.000000000000000000, 0.000000000000000000, 27.50000000000000000 ) ) ;
#36913=CARTESIAN_POINT ( 'NONE',  ( -105.5599775193885392, -56.84101280297493020, 32.50000000000000711 ) ) ;
#36923=CARTESIAN_POINT ( 'NONE',  ( -101.4249800177817207, -31.43204461043823272, 27.50000000000000000 ) ) ;
#36925=EDGE_CURVE ( 'NONE', #23651, #18582, #8798, .T. ) ;
#36930=VECTOR ( 'NONE', #23366, 1000.000000000000000 ) ;
#36936=EDGE_LOOP ( 'NONE', ( #18080, #31585, #29045, #29016 ) ) ;
#36954=VERTEX_POINT ( 'NONE', #2360 ) ;
#36973=AXIS2_PLACEMENT_3D ( 'NONE', #24936, #22298, #21927 ) ;
#37011=CARTESIAN_POINT ( 'NONE',  ( 5.089798887113564874, 119.6083602675371651, 27.49998799999999477 ) ) ;
#37014=VERTEX_POINT ( 'NONE', #19240 ) ;
#37019=CARTESIAN_POINT ( 'NONE',  ( -37.50000000000000000, 103.4105893997321743, 32.50000000000000000 ) ) ;
#37026=DIRECTION ( 'NONE',  ( 1.000000000000000000, 0.000000000000000000, 0.000000000000000000 ) ) ;
#37034=ORIENTED_EDGE ( 'NONE', *, *, #23789, .T. ) ;
#37047=CARTESIAN_POINT ( 'NONE',  ( 145.0000000000000568, -5.056524707326808249E-13, 32.50000000000000000 ) ) ;
#37052=ORIENTED_EDGE ( 'NONE', *, *, #15282, .F. ) ;
#37055=DIRECTION ( 'NONE',  ( 1.000000000000000000, 0.000000000000000000, 0.000000000000000000 ) ) ;
#37057=CARTESIAN_POINT ( 'NONE',  ( 139.0000000000000284, -5.056524707326808249E-13, 27.50000000000000000 ) ) ;
#37066=VERTEX_POINT ( 'NONE', #6454 ) ;
#37090=ADVANCED_FACE ( 'NONE', ( #252 ), #3461, .F. ) ;
#37096=AXIS2_PLACEMENT_3D ( 'NONE', #11100, #1932, #24817 ) ;
ENDSEC;
END-ISO-10303-21;
